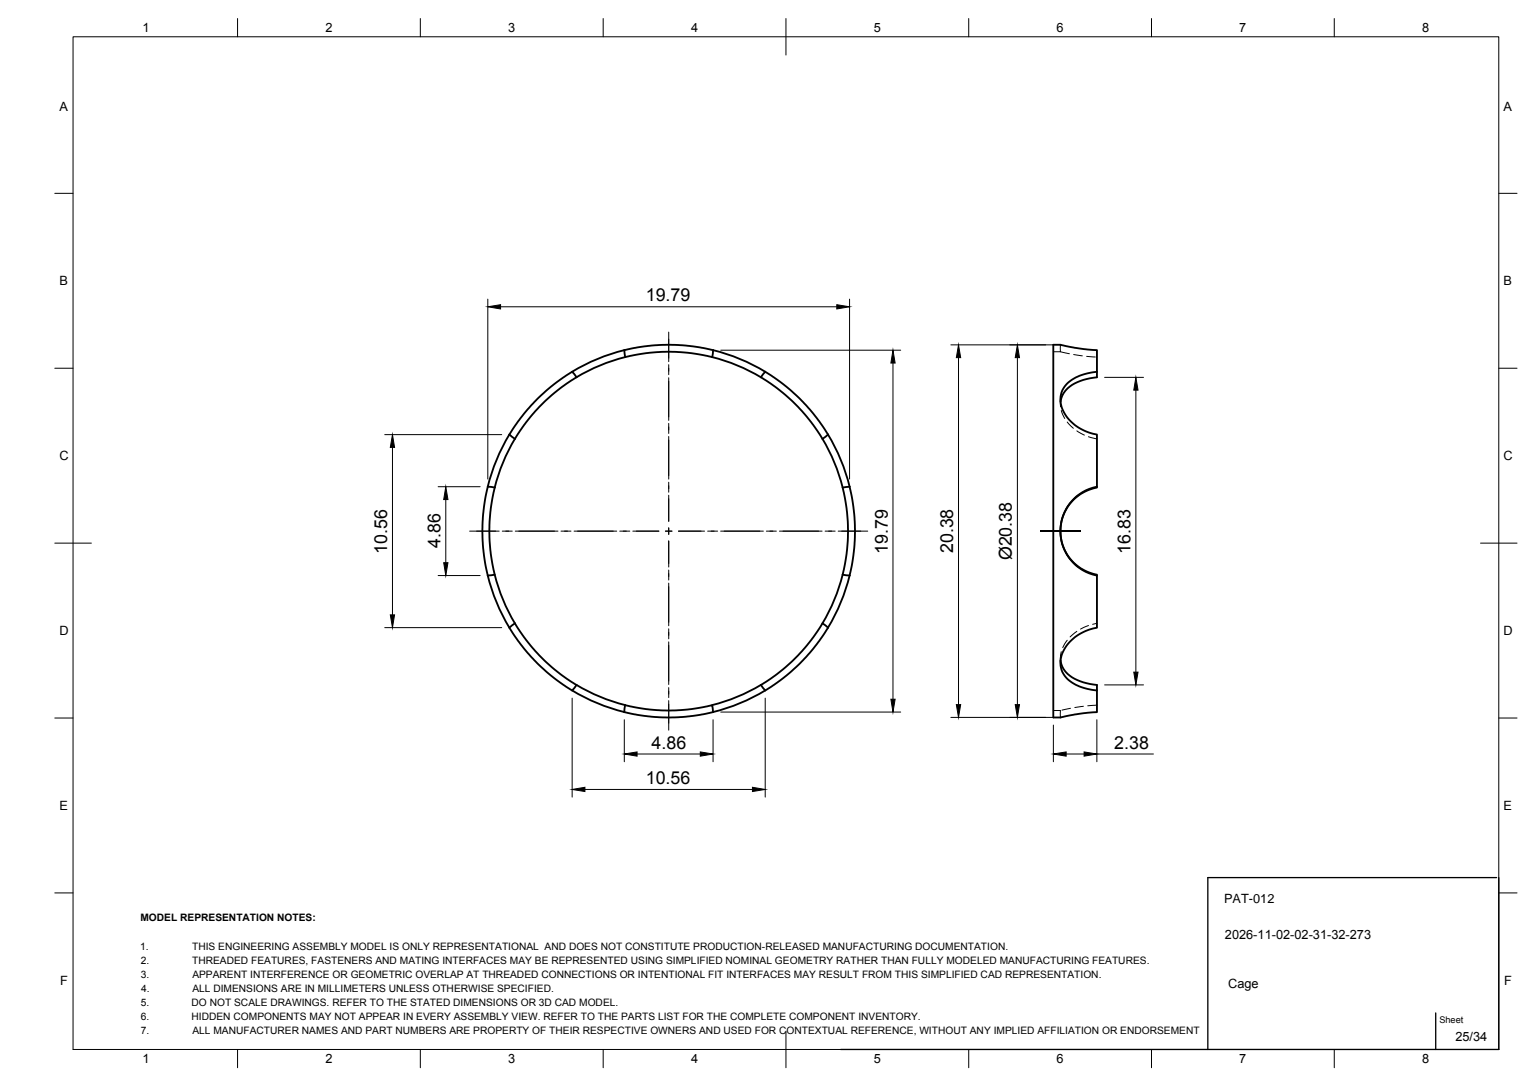
ISO-10303-21;
HEADER;
/* Generated by software containing ST-Developer
 * from STEP Tools, Inc. (www.steptools.com) 
 */

FILE_DESCRIPTION(
/* description */ ('Belt tensioner idler arm'),
/* implementation_level */ '2;1');

FILE_NAME(
/* name */ 'Cage.step',
/* time_stamp */ '2026-10-28T03:22:15-07:00',
/* author */ (''),
/* organization */ (''),
/* preprocessor_version */ 'ST-DEVELOPER v20.2',
/* originating_system */ 'Autodesk Translation Framework v15.17.0.0',
/* authorisation */ '');

FILE_SCHEMA (('AUTOMOTIVE_DESIGN { 1 0 10303 214 3 1 1 }'));
ENDSEC;

DATA;
#10=MECHANICAL_DESIGN_GEOMETRIC_PRESENTATION_REPRESENTATION('',(#475),#12779);
#263=SPHERICAL_SURFACE('',#7025,0.247676);
#264=SPHERICAL_SURFACE('',#7041,0.247676);
#265=SPHERICAL_SURFACE('',#7046,0.247676);
#266=SPHERICAL_SURFACE('',#7051,0.247676);
#267=SPHERICAL_SURFACE('',#7056,0.247676);
#268=SPHERICAL_SURFACE('',#7061,0.247676);
#269=SPHERICAL_SURFACE('',#7066,0.247676);
#270=SPHERICAL_SURFACE('',#7074,0.247676);
#334=B_SPLINE_CURVE_WITH_KNOTS('',3,(#11192,#11193,#11194,#11195,#11196,
#11197,#11198,#11199,#11200,#11201,#11202,#11203,#11204,#11205,#11206,#11207,
#11208,#11209,#11210,#11211,#11212,#11213),.UNSPECIFIED.,.F.,.F.,(4,2,2,
2,2,2,2,2,2,2,4),(0.0473477652366656,0.126350602536658,0.189525903804987,
0.252701205073317,0.313298422430275,0.373895639787233,0.434492857144191,
0.495090074501149,0.558265375769478,0.621440677037807,0.7004435143378),
 .UNSPECIFIED.);
#335=B_SPLINE_CURVE_WITH_KNOTS('',3,(#11217,#11218,#11219,#11220,#11221,
#11222,#11223,#11224,#11225,#11226,#11227,#11228,#11229,#11230,#11231,#11232,
#11233,#11234,#11235,#11236,#11237,#11238),.UNSPECIFIED.,.F.,.F.,(4,2,2,
2,2,2,2,2,2,2,4),(0.0464897534940957,0.0852567806515119,0.170513561303024,
0.246687263103517,0.308657850341199,0.370628437578881,0.432599024816563,
0.494569612054245,0.570743313854739,0.656000094506251,0.694767121663666),
 .UNSPECIFIED.);
#336=B_SPLINE_CURVE_WITH_KNOTS('',3,(#11244,#11245,#11246,#11247,#11248,
#11249,#11250,#11251,#11252,#11253,#11254,#11255,#11256,#11257,#11258,#11259,
#11260,#11261,#11262,#11263,#11264,#11265),.UNSPECIFIED.,.F.,.F.,(4,2,2,
2,2,2,2,2,2,2,4),(0.0464897534940957,0.0852567806515118,0.170513561303024,
0.246687263103517,0.308657850341199,0.370628437578881,0.432599024816563,
0.494569612054245,0.570743313854738,0.65600009450625,0.694767121663666),
 .UNSPECIFIED.);
#337=B_SPLINE_CURVE_WITH_KNOTS('',3,(#11269,#11270,#11271,#11272,#11273,
#11274,#11275,#11276,#11277,#11278,#11279,#11280,#11281,#11282,#11283,#11284,
#11285,#11286,#11287,#11288,#11289,#11290),.UNSPECIFIED.,.F.,.F.,(4,2,2,
2,2,2,2,2,2,2,4),(0.0464897534940957,0.0852567806515119,0.170513561303024,
0.246687263103517,0.308657850341199,0.370628437578881,0.432599024816563,
0.494569612054245,0.570743313854739,0.656000094506251,0.694767121663666),
 .UNSPECIFIED.);
#338=B_SPLINE_CURVE_WITH_KNOTS('',3,(#11294,#11295,#11296,#11297,#11298,
#11299,#11300,#11301,#11302,#11303,#11304,#11305),.UNSPECIFIED.,.F.,.F.,
(4,2,2,2,2,4),(0.0464897534940957,0.0852567806515119,0.170513561303024,
0.246687263103517,0.308657850341199,0.370628437578881),.UNSPECIFIED.);
#339=B_SPLINE_CURVE_WITH_KNOTS('',3,(#11310,#11311,#11312,#11313,#11314,
#11315,#11316,#11317,#11318,#11319,#11320,#11321),.UNSPECIFIED.,.F.,.F.,
(4,2,2,2,2,4),(0.370628437578881,0.432599024816563,0.494569612054245,0.570743313854738,
0.65600009450625,0.694767121663666),.UNSPECIFIED.);
#340=B_SPLINE_CURVE_WITH_KNOTS('',3,(#11325,#11326,#11327,#11328,#11329,
#11330,#11331,#11332,#11333,#11334,#11335,#11336,#11337,#11338,#11339,#11340,
#11341,#11342,#11343,#11344,#11345,#11346),.UNSPECIFIED.,.F.,.F.,(4,2,2,
2,2,2,2,2,2,2,4),(0.0464897534940957,0.0852567806515121,0.170513561303024,
0.246687263103518,0.308657850341199,0.370628437578881,0.432599024816563,
0.494569612054245,0.570743313854738,0.65600009450625,0.694767121663666),
 .UNSPECIFIED.);
#341=B_SPLINE_CURVE_WITH_KNOTS('',3,(#11350,#11351,#11352,#11353,#11354,
#11355,#11356,#11357,#11358,#11359,#11360,#11361,#11362,#11363,#11364,#11365,
#11366,#11367,#11368,#11369,#11370,#11371),.UNSPECIFIED.,.F.,.F.,(4,2,2,
2,2,2,2,2,2,2,4),(0.0464897534940957,0.0852567806515119,0.170513561303024,
0.246687263103517,0.308657850341199,0.370628437578881,0.432599024816563,
0.494569612054245,0.570743313854738,0.65600009450625,0.694767121663667),
 .UNSPECIFIED.);
#342=B_SPLINE_CURVE_WITH_KNOTS('',3,(#11375,#11376,#11377,#11378,#11379,
#11380,#11381,#11382,#11383,#11384,#11385,#11386,#11387,#11388,#11389,#11390,
#11391,#11392,#11393,#11394,#11395,#11396),.UNSPECIFIED.,.F.,.F.,(4,2,2,
2,2,2,2,2,2,2,4),(0.0464897534940957,0.0852567806515119,0.170513561303024,
0.246687263103517,0.308657850341199,0.370628437578881,0.432599024816563,
0.494569612054245,0.570743313854738,0.65600009450625,0.694767121663666),
 .UNSPECIFIED.);
#343=B_SPLINE_CURVE_WITH_KNOTS('',3,(#11400,#11401,#11402,#11403,#11404,
#11405,#11406,#11407,#11408,#11409,#11410,#11411,#11412,#11413,#11414,#11415,
#11416,#11417,#11418,#11419,#11420,#11421),.UNSPECIFIED.,.F.,.F.,(4,2,2,
2,2,2,2,2,2,2,4),(0.0464897534940957,0.0852567806515119,0.170513561303024,
0.246687263103517,0.308657850341199,0.370628437578881,0.432599024816563,
0.494569612054245,0.570743313854739,0.656000094506251,0.694767121663667),
 .UNSPECIFIED.);
#344=B_SPLINE_CURVE_WITH_KNOTS('',3,(#11429,#11430,#11431,#11432,#11433,
#11434,#11435,#11436,#11437,#11438,#11439,#11440,#11441,#11442,#11443,#11444,
#11445,#11446,#11447,#11448,#11449,#11450),.UNSPECIFIED.,.F.,.F.,(4,2,2,
2,2,2,2,2,2,2,4),(0.0473477652366656,0.126350602536658,0.189525903804987,
0.252701205073316,0.313298422430274,0.373895639787232,0.434492857144191,
0.495090074501149,0.558265375769478,0.621440677037807,0.7004435143378),
 .UNSPECIFIED.);
#345=B_SPLINE_CURVE_WITH_KNOTS('',3,(#11458,#11459,#11460,#11461,#11462,
#11463,#11464,#11465,#11466,#11467,#11468,#11469,#11470,#11471,#11472,#11473,
#11474,#11475,#11476,#11477,#11478,#11479),.UNSPECIFIED.,.F.,.F.,(4,2,2,
2,2,2,2,2,2,2,4),(0.0473477652366656,0.126350602536658,0.189525903804987,
0.252701205073317,0.313298422430275,0.373895639787233,0.434492857144191,
0.495090074501149,0.558265375769478,0.621440677037807,0.7004435143378),
 .UNSPECIFIED.);
#346=B_SPLINE_CURVE_WITH_KNOTS('',3,(#11488,#11489,#11490,#11491,#11492,
#11493,#11494,#11495,#11496,#11497,#11498,#11499),.UNSPECIFIED.,.F.,.F.,
(4,2,2,2,2,4),(0.0473477652366656,0.126350602536658,0.189525903804987,0.252701205073316,
0.313298422430275,0.373895639787233),.UNSPECIFIED.);
#347=B_SPLINE_CURVE_WITH_KNOTS('',3,(#11501,#11502,#11503,#11504,#11505,
#11506,#11507,#11508,#11509,#11510,#11511,#11512),.UNSPECIFIED.,.F.,.F.,
(4,2,2,2,2,4),(0.373895639787233,0.434492857144191,0.495090074501149,0.558265375769478,
0.621440677037807,0.7004435143378),.UNSPECIFIED.);
#348=B_SPLINE_CURVE_WITH_KNOTS('',3,(#11519,#11520,#11521,#11522,#11523,
#11524,#11525,#11526,#11527,#11528,#11529,#11530,#11531,#11532,#11533,#11534,
#11535,#11536,#11537,#11538,#11539,#11540),.UNSPECIFIED.,.F.,.F.,(4,2,2,
2,2,2,2,2,2,2,4),(0.0473477652366656,0.126350602536658,0.189525903804987,
0.252701205073316,0.313298422430275,0.373895639787233,0.434492857144191,
0.495090074501149,0.558265375769478,0.621440677037807,0.7004435143378),
 .UNSPECIFIED.);
#349=B_SPLINE_CURVE_WITH_KNOTS('',3,(#11548,#11549,#11550,#11551,#11552,
#11553,#11554,#11555,#11556,#11557,#11558,#11559,#11560,#11561,#11562,#11563,
#11564,#11565,#11566,#11567,#11568,#11569),.UNSPECIFIED.,.F.,.F.,(4,2,2,
2,2,2,2,2,2,2,4),(0.0473477652366656,0.126350602536658,0.189525903804987,
0.252701205073317,0.313298422430275,0.373895639787233,0.434492857144191,
0.495090074501149,0.558265375769478,0.621440677037807,0.7004435143378),
 .UNSPECIFIED.);
#350=B_SPLINE_CURVE_WITH_KNOTS('',3,(#11577,#11578,#11579,#11580,#11581,
#11582,#11583,#11584,#11585,#11586,#11587,#11588,#11589,#11590,#11591,#11592,
#11593,#11594,#11595,#11596,#11597,#11598),.UNSPECIFIED.,.F.,.F.,(4,2,2,
2,2,2,2,2,2,2,4),(0.0473477652366656,0.126350602536658,0.189525903804987,
0.252701205073316,0.313298422430275,0.373895639787233,0.434492857144191,
0.495090074501149,0.558265375769478,0.621440677037807,0.7004435143378),
 .UNSPECIFIED.);
#351=B_SPLINE_CURVE_WITH_KNOTS('',3,(#11607,#11608,#11609,#11610,#11611,
#11612,#11613,#11614,#11615,#11616,#11617,#11618,#11619,#11620,#11621,#11622,
#11623,#11624,#11625,#11626,#11627,#11628),.UNSPECIFIED.,.F.,.F.,(4,2,2,
2,2,2,2,2,2,2,4),(0.0473477652366656,0.126350602536658,0.189525903804987,
0.252701205073317,0.313298422430275,0.373895639787233,0.434492857144191,
0.495090074501149,0.558265375769478,0.621440677037807,0.7004435143378),
 .UNSPECIFIED.);
#400=SHAPE_REPRESENTATION_RELATIONSHIP('SRR','None',#12948,#434);
#434=ADVANCED_BREP_SHAPE_REPRESENTATION('',(#515),#12765);
#475=STYLED_ITEM('',(#13184),#515);
#515=MANIFOLD_SOLID_BREP('Continuous crown cage',#6211);
#631=FACE_BOUND('',#1536,.T.);
#769=PLANE('',#7038);
#770=PLANE('',#7043);
#771=PLANE('',#7048);
#772=PLANE('',#7053);
#773=PLANE('',#7058);
#774=PLANE('',#7063);
#775=PLANE('',#7072);
#776=PLANE('',#7076);
#777=PLANE('',#7077);
#1047=FACE_OUTER_BOUND('',#1518,.T.);
#1048=FACE_OUTER_BOUND('',#1519,.T.);
#1049=FACE_OUTER_BOUND('',#1520,.T.);
#1050=FACE_OUTER_BOUND('',#1521,.T.);
#1051=FACE_OUTER_BOUND('',#1522,.T.);
#1052=FACE_OUTER_BOUND('',#1523,.T.);
#1053=FACE_OUTER_BOUND('',#1524,.T.);
#1054=FACE_OUTER_BOUND('',#1525,.T.);
#1055=FACE_OUTER_BOUND('',#1526,.T.);
#1056=FACE_OUTER_BOUND('',#1527,.T.);
#1057=FACE_OUTER_BOUND('',#1528,.T.);
#1058=FACE_OUTER_BOUND('',#1529,.T.);
#1059=FACE_OUTER_BOUND('',#1530,.T.);
#1060=FACE_OUTER_BOUND('',#1531,.T.);
#1061=FACE_OUTER_BOUND('',#1532,.T.);
#1062=FACE_OUTER_BOUND('',#1533,.T.);
#1063=FACE_OUTER_BOUND('',#1534,.T.);
#1064=FACE_OUTER_BOUND('',#1535,.T.);
#1065=FACE_OUTER_BOUND('',#1537,.T.);
#1518=EDGE_LOOP('',(#4940,#4941,#4942,#4943));
#1519=EDGE_LOOP('',(#4944,#4945,#4946,#4947,#4948,#4949,#4950,#4951,#4952,
#4953,#4954,#4955,#4956,#4957,#4958,#4959,#4960,#4961,#4962,#4963));
#1520=EDGE_LOOP('',(#4964,#4965,#4966,#4967));
#1521=EDGE_LOOP('',(#4968,#4969,#4970,#4971));
#1522=EDGE_LOOP('',(#4972,#4973,#4974,#4975));
#1523=EDGE_LOOP('',(#4976,#4977,#4978,#4979));
#1524=EDGE_LOOP('',(#4980,#4981,#4982,#4983));
#1525=EDGE_LOOP('',(#4984,#4985,#4986,#4987,#4988,#4989));
#1526=EDGE_LOOP('',(#4990,#4991,#4992,#4993));
#1527=EDGE_LOOP('',(#4994,#4995,#4996,#4997));
#1528=EDGE_LOOP('',(#4998,#4999,#5000,#5001));
#1529=EDGE_LOOP('',(#5002,#5003,#5004,#5005));
#1530=EDGE_LOOP('',(#5006,#5007,#5008,#5009));
#1531=EDGE_LOOP('',(#5010,#5011,#5012,#5013));
#1532=EDGE_LOOP('',(#5014,#5015,#5016,#5017,#5018,#5019,#5020,#5021,#5022,
#5023,#5024,#5025,#5026,#5027,#5028,#5029,#5030,#5031,#5032,#5033));
#1533=EDGE_LOOP('',(#5034,#5035,#5036,#5037));
#1534=EDGE_LOOP('',(#5038,#5039,#5040,#5041));
#1535=EDGE_LOOP('',(#5042));
#1536=EDGE_LOOP('',(#5043));
#1537=EDGE_LOOP('',(#5044,#5045,#5046,#5047));
#1917=LINE('',#11307,#2266);
#1918=LINE('',#11603,#2267);
#2266=VECTOR('',#8503,1.019052);
#2267=VECTOR('',#8580,0.980948);
#2592=CIRCLE('',#7026,0.243053047864041);
#2593=CIRCLE('',#7027,0.243053047864041);
#2594=CIRCLE('',#7029,1.019052);
#2595=CIRCLE('',#7030,1.019052);
#2596=CIRCLE('',#7031,1.019052);
#2597=CIRCLE('',#7032,1.019052);
#2598=CIRCLE('',#7033,1.019052);
#2599=CIRCLE('',#7034,1.019052);
#2600=CIRCLE('',#7035,1.019052);
#2601=CIRCLE('',#7036,1.019052);
#2602=CIRCLE('',#7037,1.019052);
#2603=CIRCLE('',#7039,0.980948);
#2604=CIRCLE('',#7040,0.243053047864041);
#2605=CIRCLE('',#7042,0.243053047864041);
#2606=CIRCLE('',#7044,0.980948);
#2607=CIRCLE('',#7045,0.243053047864041);
#2608=CIRCLE('',#7047,0.243053047864041);
#2609=CIRCLE('',#7049,0.980948);
#2610=CIRCLE('',#7050,0.243053047864041);
#2611=CIRCLE('',#7052,0.243053047864041);
#2612=CIRCLE('',#7054,0.980948);
#2613=CIRCLE('',#7055,0.243053047864041);
#2614=CIRCLE('',#7057,0.243053047864041);
#2615=CIRCLE('',#7059,0.980948);
#2616=CIRCLE('',#7060,0.243053047864041);
#2617=CIRCLE('',#7062,0.243053047864041);
#2618=CIRCLE('',#7064,0.980948);
#2619=CIRCLE('',#7065,0.243053047864041);
#2620=CIRCLE('',#7067,0.243053047864041);
#2621=CIRCLE('',#7069,0.980948);
#2622=CIRCLE('',#7070,0.980948);
#2623=CIRCLE('',#7071,0.980948);
#2624=CIRCLE('',#7073,0.243053047864041);
#2625=CIRCLE('',#7075,0.243053047864041);
#3056=VERTEX_POINT('',#11190);
#3057=VERTEX_POINT('',#11191);
#3058=VERTEX_POINT('',#11214);
#3059=VERTEX_POINT('',#11216);
#3060=VERTEX_POINT('',#11241);
#3061=VERTEX_POINT('',#11243);
#3062=VERTEX_POINT('',#11266);
#3063=VERTEX_POINT('',#11268);
#3064=VERTEX_POINT('',#11291);
#3065=VERTEX_POINT('',#11293);
#3066=VERTEX_POINT('',#11306);
#3067=VERTEX_POINT('',#11309);
#3068=VERTEX_POINT('',#11322);
#3069=VERTEX_POINT('',#11324);
#3070=VERTEX_POINT('',#11347);
#3071=VERTEX_POINT('',#11349);
#3072=VERTEX_POINT('',#11372);
#3073=VERTEX_POINT('',#11374);
#3074=VERTEX_POINT('',#11397);
#3075=VERTEX_POINT('',#11399);
#3076=VERTEX_POINT('',#11424);
#3077=VERTEX_POINT('',#11428);
#3078=VERTEX_POINT('',#11453);
#3079=VERTEX_POINT('',#11457);
#3080=VERTEX_POINT('',#11482);
#3081=VERTEX_POINT('',#11486);
#3082=VERTEX_POINT('',#11487);
#3083=VERTEX_POINT('',#11514);
#3084=VERTEX_POINT('',#11518);
#3085=VERTEX_POINT('',#11543);
#3086=VERTEX_POINT('',#11547);
#3087=VERTEX_POINT('',#11572);
#3088=VERTEX_POINT('',#11576);
#3089=VERTEX_POINT('',#11601);
#3090=VERTEX_POINT('',#11604);
#3091=VERTEX_POINT('',#11606);
#3725=EDGE_CURVE('',#3056,#3057,#334,.T.);
#3726=EDGE_CURVE('',#3058,#3056,#2592,.T.);
#3727=EDGE_CURVE('',#3059,#3058,#335,.T.);
#3728=EDGE_CURVE('',#3057,#3059,#2593,.T.);
#3729=EDGE_CURVE('',#3060,#3058,#2594,.T.);
#3730=EDGE_CURVE('',#3060,#3061,#336,.T.);
#3731=EDGE_CURVE('',#3062,#3061,#2595,.T.);
#3732=EDGE_CURVE('',#3062,#3063,#337,.T.);
#3733=EDGE_CURVE('',#3064,#3063,#2596,.T.);
#3734=EDGE_CURVE('',#3064,#3065,#338,.T.);
#3735=EDGE_CURVE('',#3065,#3066,#1917,.T.);
#3736=EDGE_CURVE('',#3066,#3066,#2597,.T.);
#3737=EDGE_CURVE('',#3065,#3067,#339,.T.);
#3738=EDGE_CURVE('',#3068,#3067,#2598,.T.);
#3739=EDGE_CURVE('',#3068,#3069,#340,.T.);
#3740=EDGE_CURVE('',#3070,#3069,#2599,.T.);
#3741=EDGE_CURVE('',#3070,#3071,#341,.T.);
#3742=EDGE_CURVE('',#3072,#3071,#2600,.T.);
#3743=EDGE_CURVE('',#3072,#3073,#342,.T.);
#3744=EDGE_CURVE('',#3074,#3073,#2601,.T.);
#3745=EDGE_CURVE('',#3074,#3075,#343,.T.);
#3746=EDGE_CURVE('',#3059,#3075,#2602,.T.);
#3747=EDGE_CURVE('',#3056,#3076,#2603,.T.);
#3748=EDGE_CURVE('',#3076,#3060,#2604,.T.);
#3749=EDGE_CURVE('',#3077,#3076,#344,.T.);
#3750=EDGE_CURVE('',#3061,#3077,#2605,.T.);
#3751=EDGE_CURVE('',#3077,#3078,#2606,.T.);
#3752=EDGE_CURVE('',#3078,#3062,#2607,.T.);
#3753=EDGE_CURVE('',#3079,#3078,#345,.T.);
#3754=EDGE_CURVE('',#3063,#3079,#2608,.T.);
#3755=EDGE_CURVE('',#3079,#3080,#2609,.T.);
#3756=EDGE_CURVE('',#3080,#3064,#2610,.T.);
#3757=EDGE_CURVE('',#3081,#3082,#346,.T.);
#3758=EDGE_CURVE('',#3067,#3081,#2611,.T.);
#3759=EDGE_CURVE('',#3082,#3080,#347,.T.);
#3760=EDGE_CURVE('',#3081,#3083,#2612,.T.);
#3761=EDGE_CURVE('',#3083,#3068,#2613,.T.);
#3762=EDGE_CURVE('',#3084,#3083,#348,.T.);
#3763=EDGE_CURVE('',#3069,#3084,#2614,.T.);
#3764=EDGE_CURVE('',#3084,#3085,#2615,.T.);
#3765=EDGE_CURVE('',#3085,#3070,#2616,.T.);
#3766=EDGE_CURVE('',#3086,#3085,#349,.T.);
#3767=EDGE_CURVE('',#3071,#3086,#2617,.T.);
#3768=EDGE_CURVE('',#3086,#3087,#2618,.T.);
#3769=EDGE_CURVE('',#3087,#3072,#2619,.T.);
#3770=EDGE_CURVE('',#3088,#3087,#350,.T.);
#3771=EDGE_CURVE('',#3073,#3088,#2620,.T.);
#3772=EDGE_CURVE('',#3089,#3089,#2621,.T.);
#3773=EDGE_CURVE('',#3089,#3082,#1918,.T.);
#3774=EDGE_CURVE('',#3090,#3057,#2622,.T.);
#3775=EDGE_CURVE('',#3090,#3091,#351,.T.);
#3776=EDGE_CURVE('',#3088,#3091,#2623,.T.);
#3777=EDGE_CURVE('',#3075,#3090,#2624,.T.);
#3778=EDGE_CURVE('',#3091,#3074,#2625,.T.);
#4940=ORIENTED_EDGE('',*,*,#3725,.F.);
#4941=ORIENTED_EDGE('',*,*,#3726,.F.);
#4942=ORIENTED_EDGE('',*,*,#3727,.F.);
#4943=ORIENTED_EDGE('',*,*,#3728,.F.);
#4944=ORIENTED_EDGE('',*,*,#3727,.T.);
#4945=ORIENTED_EDGE('',*,*,#3729,.F.);
#4946=ORIENTED_EDGE('',*,*,#3730,.T.);
#4947=ORIENTED_EDGE('',*,*,#3731,.F.);
#4948=ORIENTED_EDGE('',*,*,#3732,.T.);
#4949=ORIENTED_EDGE('',*,*,#3733,.F.);
#4950=ORIENTED_EDGE('',*,*,#3734,.T.);
#4951=ORIENTED_EDGE('',*,*,#3735,.T.);
#4952=ORIENTED_EDGE('',*,*,#3736,.F.);
#4953=ORIENTED_EDGE('',*,*,#3735,.F.);
#4954=ORIENTED_EDGE('',*,*,#3737,.T.);
#4955=ORIENTED_EDGE('',*,*,#3738,.F.);
#4956=ORIENTED_EDGE('',*,*,#3739,.T.);
#4957=ORIENTED_EDGE('',*,*,#3740,.F.);
#4958=ORIENTED_EDGE('',*,*,#3741,.T.);
#4959=ORIENTED_EDGE('',*,*,#3742,.F.);
#4960=ORIENTED_EDGE('',*,*,#3743,.T.);
#4961=ORIENTED_EDGE('',*,*,#3744,.F.);
#4962=ORIENTED_EDGE('',*,*,#3745,.T.);
#4963=ORIENTED_EDGE('',*,*,#3746,.F.);
#4964=ORIENTED_EDGE('',*,*,#3726,.T.);
#4965=ORIENTED_EDGE('',*,*,#3747,.T.);
#4966=ORIENTED_EDGE('',*,*,#3748,.T.);
#4967=ORIENTED_EDGE('',*,*,#3729,.T.);
#4968=ORIENTED_EDGE('',*,*,#3749,.F.);
#4969=ORIENTED_EDGE('',*,*,#3750,.F.);
#4970=ORIENTED_EDGE('',*,*,#3730,.F.);
#4971=ORIENTED_EDGE('',*,*,#3748,.F.);
#4972=ORIENTED_EDGE('',*,*,#3750,.T.);
#4973=ORIENTED_EDGE('',*,*,#3751,.T.);
#4974=ORIENTED_EDGE('',*,*,#3752,.T.);
#4975=ORIENTED_EDGE('',*,*,#3731,.T.);
#4976=ORIENTED_EDGE('',*,*,#3753,.F.);
#4977=ORIENTED_EDGE('',*,*,#3754,.F.);
#4978=ORIENTED_EDGE('',*,*,#3732,.F.);
#4979=ORIENTED_EDGE('',*,*,#3752,.F.);
#4980=ORIENTED_EDGE('',*,*,#3754,.T.);
#4981=ORIENTED_EDGE('',*,*,#3755,.T.);
#4982=ORIENTED_EDGE('',*,*,#3756,.T.);
#4983=ORIENTED_EDGE('',*,*,#3733,.T.);
#4984=ORIENTED_EDGE('',*,*,#3757,.F.);
#4985=ORIENTED_EDGE('',*,*,#3758,.F.);
#4986=ORIENTED_EDGE('',*,*,#3737,.F.);
#4987=ORIENTED_EDGE('',*,*,#3734,.F.);
#4988=ORIENTED_EDGE('',*,*,#3756,.F.);
#4989=ORIENTED_EDGE('',*,*,#3759,.F.);
#4990=ORIENTED_EDGE('',*,*,#3758,.T.);
#4991=ORIENTED_EDGE('',*,*,#3760,.T.);
#4992=ORIENTED_EDGE('',*,*,#3761,.T.);
#4993=ORIENTED_EDGE('',*,*,#3738,.T.);
#4994=ORIENTED_EDGE('',*,*,#3762,.F.);
#4995=ORIENTED_EDGE('',*,*,#3763,.F.);
#4996=ORIENTED_EDGE('',*,*,#3739,.F.);
#4997=ORIENTED_EDGE('',*,*,#3761,.F.);
#4998=ORIENTED_EDGE('',*,*,#3763,.T.);
#4999=ORIENTED_EDGE('',*,*,#3764,.T.);
#5000=ORIENTED_EDGE('',*,*,#3765,.T.);
#5001=ORIENTED_EDGE('',*,*,#3740,.T.);
#5002=ORIENTED_EDGE('',*,*,#3766,.F.);
#5003=ORIENTED_EDGE('',*,*,#3767,.F.);
#5004=ORIENTED_EDGE('',*,*,#3741,.F.);
#5005=ORIENTED_EDGE('',*,*,#3765,.F.);
#5006=ORIENTED_EDGE('',*,*,#3767,.T.);
#5007=ORIENTED_EDGE('',*,*,#3768,.T.);
#5008=ORIENTED_EDGE('',*,*,#3769,.T.);
#5009=ORIENTED_EDGE('',*,*,#3742,.T.);
#5010=ORIENTED_EDGE('',*,*,#3743,.F.);
#5011=ORIENTED_EDGE('',*,*,#3769,.F.);
#5012=ORIENTED_EDGE('',*,*,#3770,.F.);
#5013=ORIENTED_EDGE('',*,*,#3771,.F.);
#5014=ORIENTED_EDGE('',*,*,#3772,.F.);
#5015=ORIENTED_EDGE('',*,*,#3773,.T.);
#5016=ORIENTED_EDGE('',*,*,#3759,.T.);
#5017=ORIENTED_EDGE('',*,*,#3755,.F.);
#5018=ORIENTED_EDGE('',*,*,#3753,.T.);
#5019=ORIENTED_EDGE('',*,*,#3751,.F.);
#5020=ORIENTED_EDGE('',*,*,#3749,.T.);
#5021=ORIENTED_EDGE('',*,*,#3747,.F.);
#5022=ORIENTED_EDGE('',*,*,#3725,.T.);
#5023=ORIENTED_EDGE('',*,*,#3774,.F.);
#5024=ORIENTED_EDGE('',*,*,#3775,.T.);
#5025=ORIENTED_EDGE('',*,*,#3776,.F.);
#5026=ORIENTED_EDGE('',*,*,#3770,.T.);
#5027=ORIENTED_EDGE('',*,*,#3768,.F.);
#5028=ORIENTED_EDGE('',*,*,#3766,.T.);
#5029=ORIENTED_EDGE('',*,*,#3764,.F.);
#5030=ORIENTED_EDGE('',*,*,#3762,.T.);
#5031=ORIENTED_EDGE('',*,*,#3760,.F.);
#5032=ORIENTED_EDGE('',*,*,#3757,.T.);
#5033=ORIENTED_EDGE('',*,*,#3773,.F.);
#5034=ORIENTED_EDGE('',*,*,#3728,.T.);
#5035=ORIENTED_EDGE('',*,*,#3746,.T.);
#5036=ORIENTED_EDGE('',*,*,#3777,.T.);
#5037=ORIENTED_EDGE('',*,*,#3774,.T.);
#5038=ORIENTED_EDGE('',*,*,#3745,.F.);
#5039=ORIENTED_EDGE('',*,*,#3778,.F.);
#5040=ORIENTED_EDGE('',*,*,#3775,.F.);
#5041=ORIENTED_EDGE('',*,*,#3777,.F.);
#5042=ORIENTED_EDGE('',*,*,#3736,.T.);
#5043=ORIENTED_EDGE('',*,*,#3772,.T.);
#5044=ORIENTED_EDGE('',*,*,#3771,.T.);
#5045=ORIENTED_EDGE('',*,*,#3776,.T.);
#5046=ORIENTED_EDGE('',*,*,#3778,.T.);
#5047=ORIENTED_EDGE('',*,*,#3744,.T.);
#5740=CYLINDRICAL_SURFACE('',#7028,1.019052);
#5741=CYLINDRICAL_SURFACE('',#7068,0.980948);
#6024=ADVANCED_FACE('',(#1047),#263,.F.);
#6025=ADVANCED_FACE('',(#1048),#5740,.T.);
#6026=ADVANCED_FACE('',(#1049),#769,.T.);
#6027=ADVANCED_FACE('',(#1050),#264,.F.);
#6028=ADVANCED_FACE('',(#1051),#770,.T.);
#6029=ADVANCED_FACE('',(#1052),#265,.F.);
#6030=ADVANCED_FACE('',(#1053),#771,.T.);
#6031=ADVANCED_FACE('',(#1054),#266,.F.);
#6032=ADVANCED_FACE('',(#1055),#772,.T.);
#6033=ADVANCED_FACE('',(#1056),#267,.F.);
#6034=ADVANCED_FACE('',(#1057),#773,.T.);
#6035=ADVANCED_FACE('',(#1058),#268,.F.);
#6036=ADVANCED_FACE('',(#1059),#774,.T.);
#6037=ADVANCED_FACE('',(#1060),#269,.F.);
#6038=ADVANCED_FACE('',(#1061),#5741,.F.);
#6039=ADVANCED_FACE('',(#1062),#775,.T.);
#6040=ADVANCED_FACE('',(#1063),#270,.F.);
#6041=ADVANCED_FACE('',(#1064,#631),#776,.T.);
#6042=ADVANCED_FACE('',(#1065),#777,.T.);
#6211=CLOSED_SHELL('',(#6024,#6025,#6026,#6027,#6028,#6029,#6030,#6031,
#6032,#6033,#6034,#6035,#6036,#6037,#6038,#6039,#6040,#6041,#6042));
#7024=AXIS2_PLACEMENT_3D('',#11188,#8487,#8488);
#7025=AXIS2_PLACEMENT_3D('',#11189,#8489,#8490);
#7026=AXIS2_PLACEMENT_3D('',#11215,#8491,#8492);
#7027=AXIS2_PLACEMENT_3D('',#11239,#8493,#8494);
#7028=AXIS2_PLACEMENT_3D('',#11240,#8495,#8496);
#7029=AXIS2_PLACEMENT_3D('',#11242,#8497,#8498);
#7030=AXIS2_PLACEMENT_3D('',#11267,#8499,#8500);
#7031=AXIS2_PLACEMENT_3D('',#11292,#8501,#8502);
#7032=AXIS2_PLACEMENT_3D('',#11308,#8504,#8505);
#7033=AXIS2_PLACEMENT_3D('',#11323,#8506,#8507);
#7034=AXIS2_PLACEMENT_3D('',#11348,#8508,#8509);
#7035=AXIS2_PLACEMENT_3D('',#11373,#8510,#8511);
#7036=AXIS2_PLACEMENT_3D('',#11398,#8512,#8513);
#7037=AXIS2_PLACEMENT_3D('',#11422,#8514,#8515);
#7038=AXIS2_PLACEMENT_3D('',#11423,#8516,#8517);
#7039=AXIS2_PLACEMENT_3D('',#11425,#8518,#8519);
#7040=AXIS2_PLACEMENT_3D('',#11426,#8520,#8521);
#7041=AXIS2_PLACEMENT_3D('',#11427,#8522,#8523);
#7042=AXIS2_PLACEMENT_3D('',#11451,#8524,#8525);
#7043=AXIS2_PLACEMENT_3D('',#11452,#8526,#8527);
#7044=AXIS2_PLACEMENT_3D('',#11454,#8528,#8529);
#7045=AXIS2_PLACEMENT_3D('',#11455,#8530,#8531);
#7046=AXIS2_PLACEMENT_3D('',#11456,#8532,#8533);
#7047=AXIS2_PLACEMENT_3D('',#11480,#8534,#8535);
#7048=AXIS2_PLACEMENT_3D('',#11481,#8536,#8537);
#7049=AXIS2_PLACEMENT_3D('',#11483,#8538,#8539);
#7050=AXIS2_PLACEMENT_3D('',#11484,#8540,#8541);
#7051=AXIS2_PLACEMENT_3D('',#11485,#8542,#8543);
#7052=AXIS2_PLACEMENT_3D('',#11500,#8544,#8545);
#7053=AXIS2_PLACEMENT_3D('',#11513,#8546,#8547);
#7054=AXIS2_PLACEMENT_3D('',#11515,#8548,#8549);
#7055=AXIS2_PLACEMENT_3D('',#11516,#8550,#8551);
#7056=AXIS2_PLACEMENT_3D('',#11517,#8552,#8553);
#7057=AXIS2_PLACEMENT_3D('',#11541,#8554,#8555);
#7058=AXIS2_PLACEMENT_3D('',#11542,#8556,#8557);
#7059=AXIS2_PLACEMENT_3D('',#11544,#8558,#8559);
#7060=AXIS2_PLACEMENT_3D('',#11545,#8560,#8561);
#7061=AXIS2_PLACEMENT_3D('',#11546,#8562,#8563);
#7062=AXIS2_PLACEMENT_3D('',#11570,#8564,#8565);
#7063=AXIS2_PLACEMENT_3D('',#11571,#8566,#8567);
#7064=AXIS2_PLACEMENT_3D('',#11573,#8568,#8569);
#7065=AXIS2_PLACEMENT_3D('',#11574,#8570,#8571);
#7066=AXIS2_PLACEMENT_3D('',#11575,#8572,#8573);
#7067=AXIS2_PLACEMENT_3D('',#11599,#8574,#8575);
#7068=AXIS2_PLACEMENT_3D('',#11600,#8576,#8577);
#7069=AXIS2_PLACEMENT_3D('',#11602,#8578,#8579);
#7070=AXIS2_PLACEMENT_3D('',#11605,#8581,#8582);
#7071=AXIS2_PLACEMENT_3D('',#11629,#8583,#8584);
#7072=AXIS2_PLACEMENT_3D('',#11630,#8585,#8586);
#7073=AXIS2_PLACEMENT_3D('',#11631,#8587,#8588);
#7074=AXIS2_PLACEMENT_3D('',#11632,#8589,#8590);
#7075=AXIS2_PLACEMENT_3D('',#11633,#8591,#8592);
#7076=AXIS2_PLACEMENT_3D('',#11634,#8593,#8594);
#7077=AXIS2_PLACEMENT_3D('',#11635,#8595,#8596);
#8487=DIRECTION('axis',(0.,0.,1.));
#8488=DIRECTION('refdir',(1.,0.,0.));
#8489=DIRECTION('center_axis',(0.,0.,1.));
#8490=DIRECTION('ref_axis',(1.,0.,0.));
#8491=DIRECTION('center_axis',(0.,-1.,0.));
#8492=DIRECTION('ref_axis',(0.,0.,-1.));
#8493=DIRECTION('center_axis',(0.,-1.,0.));
#8494=DIRECTION('ref_axis',(0.,0.,-1.));
#8495=DIRECTION('center_axis',(0.,1.,0.));
#8496=DIRECTION('ref_axis',(1.,0.,0.));
#8497=DIRECTION('center_axis',(0.,1.,0.));
#8498=DIRECTION('ref_axis',(1.,0.,0.));
#8499=DIRECTION('center_axis',(0.,1.,0.));
#8500=DIRECTION('ref_axis',(1.,0.,0.));
#8501=DIRECTION('center_axis',(0.,1.,0.));
#8502=DIRECTION('ref_axis',(1.,0.,0.));
#8503=DIRECTION('',(0.,-1.,0.));
#8504=DIRECTION('center_axis',(0.,-1.,0.));
#8505=DIRECTION('ref_axis',(1.,0.,0.));
#8506=DIRECTION('center_axis',(0.,1.,0.));
#8507=DIRECTION('ref_axis',(1.,0.,0.));
#8508=DIRECTION('center_axis',(0.,1.,0.));
#8509=DIRECTION('ref_axis',(1.,0.,0.));
#8510=DIRECTION('center_axis',(0.,1.,0.));
#8511=DIRECTION('ref_axis',(1.,0.,0.));
#8512=DIRECTION('center_axis',(0.,1.,0.));
#8513=DIRECTION('ref_axis',(1.,0.,0.));
#8514=DIRECTION('center_axis',(0.,1.,0.));
#8515=DIRECTION('ref_axis',(1.,0.,0.));
#8516=DIRECTION('center_axis',(0.,1.,0.));
#8517=DIRECTION('ref_axis',(1.,0.,0.));
#8518=DIRECTION('center_axis',(0.,-1.,0.));
#8519=DIRECTION('ref_axis',(1.,0.,0.));
#8520=DIRECTION('center_axis',(0.,-1.,0.));
#8521=DIRECTION('ref_axis',(0.,0.,-1.));
#8522=DIRECTION('center_axis',(6.12323399573677E-17,0.,1.));
#8523=DIRECTION('ref_axis',(1.,0.,0.));
#8524=DIRECTION('center_axis',(0.,-1.,0.));
#8525=DIRECTION('ref_axis',(0.,0.,-1.));
#8526=DIRECTION('center_axis',(0.,1.,0.));
#8527=DIRECTION('ref_axis',(1.,0.,0.));
#8528=DIRECTION('center_axis',(0.,-1.,0.));
#8529=DIRECTION('ref_axis',(1.,0.,0.));
#8530=DIRECTION('center_axis',(0.,-1.,0.));
#8531=DIRECTION('ref_axis',(0.,0.,-1.));
#8532=DIRECTION('center_axis',(0.,0.,1.));
#8533=DIRECTION('ref_axis',(1.,0.,0.));
#8534=DIRECTION('center_axis',(0.,-1.,0.));
#8535=DIRECTION('ref_axis',(0.,0.,-1.));
#8536=DIRECTION('center_axis',(0.,1.,0.));
#8537=DIRECTION('ref_axis',(1.,0.,0.));
#8538=DIRECTION('center_axis',(0.,-1.,0.));
#8539=DIRECTION('ref_axis',(1.,0.,0.));
#8540=DIRECTION('center_axis',(0.,-1.,0.));
#8541=DIRECTION('ref_axis',(0.,0.,-1.));
#8542=DIRECTION('center_axis',(0.,0.,1.));
#8543=DIRECTION('ref_axis',(1.,0.,0.));
#8544=DIRECTION('center_axis',(0.,-1.,0.));
#8545=DIRECTION('ref_axis',(0.,0.,-1.));
#8546=DIRECTION('center_axis',(0.,1.,0.));
#8547=DIRECTION('ref_axis',(1.,0.,0.));
#8548=DIRECTION('center_axis',(0.,-1.,0.));
#8549=DIRECTION('ref_axis',(1.,0.,0.));
#8550=DIRECTION('center_axis',(0.,-1.,0.));
#8551=DIRECTION('ref_axis',(0.,0.,-1.));
#8552=DIRECTION('center_axis',(0.,0.,1.));
#8553=DIRECTION('ref_axis',(1.,0.,0.));
#8554=DIRECTION('center_axis',(0.,-1.,0.));
#8555=DIRECTION('ref_axis',(0.,0.,-1.));
#8556=DIRECTION('center_axis',(0.,1.,0.));
#8557=DIRECTION('ref_axis',(1.,0.,0.));
#8558=DIRECTION('center_axis',(0.,-1.,0.));
#8559=DIRECTION('ref_axis',(1.,0.,0.));
#8560=DIRECTION('center_axis',(0.,-1.,0.));
#8561=DIRECTION('ref_axis',(0.,0.,-1.));
#8562=DIRECTION('center_axis',(6.12323399573676E-17,0.,1.));
#8563=DIRECTION('ref_axis',(1.,0.,0.));
#8564=DIRECTION('center_axis',(0.,-1.,0.));
#8565=DIRECTION('ref_axis',(0.,0.,-1.));
#8566=DIRECTION('center_axis',(0.,1.,0.));
#8567=DIRECTION('ref_axis',(1.,0.,0.));
#8568=DIRECTION('center_axis',(0.,-1.,0.));
#8569=DIRECTION('ref_axis',(1.,0.,0.));
#8570=DIRECTION('center_axis',(0.,-1.,0.));
#8571=DIRECTION('ref_axis',(0.,0.,-1.));
#8572=DIRECTION('center_axis',(0.,0.,1.));
#8573=DIRECTION('ref_axis',(1.,0.,0.));
#8574=DIRECTION('center_axis',(0.,-1.,0.));
#8575=DIRECTION('ref_axis',(0.,0.,-1.));
#8576=DIRECTION('center_axis',(0.,1.,0.));
#8577=DIRECTION('ref_axis',(1.,0.,0.));
#8578=DIRECTION('center_axis',(0.,1.,0.));
#8579=DIRECTION('ref_axis',(1.,0.,0.));
#8580=DIRECTION('',(0.,1.,0.));
#8581=DIRECTION('center_axis',(0.,-1.,0.));
#8582=DIRECTION('ref_axis',(1.,0.,0.));
#8583=DIRECTION('center_axis',(0.,-1.,0.));
#8584=DIRECTION('ref_axis',(1.,0.,0.));
#8585=DIRECTION('center_axis',(0.,1.,0.));
#8586=DIRECTION('ref_axis',(1.,0.,0.));
#8587=DIRECTION('center_axis',(0.,-1.,0.));
#8588=DIRECTION('ref_axis',(0.,0.,-1.));
#8589=DIRECTION('center_axis',(0.,0.,1.));
#8590=DIRECTION('ref_axis',(1.,0.,0.));
#8591=DIRECTION('center_axis',(0.,-1.,0.));
#8592=DIRECTION('ref_axis',(0.,0.,-1.));
#8593=DIRECTION('center_axis',(0.,-1.,0.));
#8594=DIRECTION('ref_axis',(-1.,0.,0.));
#8595=DIRECTION('center_axis',(0.,1.,0.));
#8596=DIRECTION('ref_axis',(1.,0.,0.));
#11188=CARTESIAN_POINT('',(0.,0.,0.));
#11189=CARTESIAN_POINT('Origin',(0.707106781186547,0.,0.707106781186548));
#11190=CARTESIAN_POINT('',(0.504455939115715,-0.04763,0.841298510752802));
#11191=CARTESIAN_POINT('',(0.841298510752802,-0.04763,0.504455939115715));
#11192=CARTESIAN_POINT('Ctrl Pts',(0.504455939115715,-0.04763,0.841298510752802));
#11193=CARTESIAN_POINT('Ctrl Pts',(0.508899795931835,-0.0740444353928835,
0.838633903678357));
#11194=CARTESIAN_POINT('Ctrl Pts',(0.517157748491652,-0.0999305678883309,
0.833661031856294));
#11195=CARTESIAN_POINT('Ctrl Pts',(0.537715343527944,-0.142345102874864,
0.820511285096538));
#11196=CARTESIAN_POINT('Ctrl Pts',(0.548874290046456,-0.159766064500479,
0.813159949759));
#11197=CARTESIAN_POINT('Ctrl Pts',(0.573915184558107,-0.190326085855194,
0.795684265985089));
#11198=CARTESIAN_POINT('Ctrl Pts',(0.587792702767295,-0.203463743702801,
0.78555112003688));
#11199=CARTESIAN_POINT('Ctrl Pts',(0.615966552324775,-0.224161999508995,
0.763642258217233));
#11200=CARTESIAN_POINT('Ctrl Pts',(0.631684198665438,-0.232861760990032,
0.750785745543687));
#11201=CARTESIAN_POINT('Ctrl Pts',(0.663382628119203,-0.244251601209411,
0.722929908501543));
#11202=CARTESIAN_POINT('Ctrl Pts',(0.679352081686668,-0.246942143572133,
0.707917883896095));
#11203=CARTESIAN_POINT('Ctrl Pts',(0.707917883896095,-0.246942143572133,
0.679352081686668));
#11204=CARTESIAN_POINT('Ctrl Pts',(0.722929908501543,-0.244251601209411,
0.663382628119203));
#11205=CARTESIAN_POINT('Ctrl Pts',(0.750785745543687,-0.232861760990032,
0.631684198665439));
#11206=CARTESIAN_POINT('Ctrl Pts',(0.763642258217232,-0.224161999508995,
0.615966552324775));
#11207=CARTESIAN_POINT('Ctrl Pts',(0.78555112003688,-0.203463743702801,
0.587792702767295));
#11208=CARTESIAN_POINT('Ctrl Pts',(0.795684265985088,-0.190326085855194,
0.573915184558108));
#11209=CARTESIAN_POINT('Ctrl Pts',(0.813159949759,-0.15976606450048,0.548874290046456));
#11210=CARTESIAN_POINT('Ctrl Pts',(0.820511285096538,-0.142345102874864,
0.537715343527944));
#11211=CARTESIAN_POINT('Ctrl Pts',(0.833661031856294,-0.099930567888331,
0.517157748491653));
#11212=CARTESIAN_POINT('Ctrl Pts',(0.838633903678357,-0.0740444353928835,
0.508899795931835));
#11213=CARTESIAN_POINT('Ctrl Pts',(0.841298510752801,-0.0476299999999999,
0.504455939115715));
#11214=CARTESIAN_POINT('',(0.528110872004958,-0.04763,0.871530771444223));
#11215=CARTESIAN_POINT('Origin',(0.707106781186547,-0.04763,0.707106781186548));
#11216=CARTESIAN_POINT('',(0.871530771444223,-0.04763,0.528110872004959));
#11217=CARTESIAN_POINT('Ctrl Pts',(0.871530771444223,-0.0476300000000001,
0.528110872004958));
#11218=CARTESIAN_POINT('Ctrl Pts',(0.87014664509073,-0.0609922781173483,
0.530395067942936));
#11219=CARTESIAN_POINT('Ctrl Pts',(0.868149331745851,-0.0742967091364493,
0.533674141594226));
#11220=CARTESIAN_POINT('Ctrl Pts',(0.85981294420286,-0.115492077056649,
0.54708917182331));
#11221=CARTESIAN_POINT('Ctrl Pts',(0.850993704737257,-0.141695629206859,
0.560922177770136));
#11222=CARTESIAN_POINT('Ctrl Pts',(0.830754510485543,-0.181890537957859,
0.590422647829571));
#11223=CARTESIAN_POINT('Ctrl Pts',(0.816896541396381,-0.201072148666545,
0.609616703125488));
#11224=CARTESIAN_POINT('Ctrl Pts',(0.792310597819928,-0.223955109275652,
0.641117951819998));
#11225=CARTESIAN_POINT('Ctrl Pts',(0.779109323683612,-0.232742381310829,
0.657208095763053));
#11226=CARTESIAN_POINT('Ctrl Pts',(0.750552691816206,-0.244234834628584,
0.68964083160521));
#11227=CARTESIAN_POINT('Ctrl Pts',(0.735185187071673,-0.246942143572133,
0.705971972091755));
#11228=CARTESIAN_POINT('Ctrl Pts',(0.705971972091754,-0.246942143572133,
0.735185187071673));
#11229=CARTESIAN_POINT('Ctrl Pts',(0.689640831605209,-0.244234834628584,
0.750552691816206));
#11230=CARTESIAN_POINT('Ctrl Pts',(0.657208095763052,-0.232742381310829,
0.779109323683612));
#11231=CARTESIAN_POINT('Ctrl Pts',(0.641117951819998,-0.223955109275652,
0.792310597819928));
#11232=CARTESIAN_POINT('Ctrl Pts',(0.609616703125487,-0.201072148666545,
0.816896541396382));
#11233=CARTESIAN_POINT('Ctrl Pts',(0.590422647829571,-0.181890537957858,
0.830754510485544));
#11234=CARTESIAN_POINT('Ctrl Pts',(0.560922177770135,-0.141695629206858,
0.850993704737257));
#11235=CARTESIAN_POINT('Ctrl Pts',(0.547089171823309,-0.115492077056649,
0.859812944202861));
#11236=CARTESIAN_POINT('Ctrl Pts',(0.533674141594226,-0.0742967091364491,
0.868149331745852));
#11237=CARTESIAN_POINT('Ctrl Pts',(0.530395067942936,-0.0609922781173483,
0.870146645090731));
#11238=CARTESIAN_POINT('Ctrl Pts',(0.528110872004958,-0.0476300000000001,
0.871530771444223));
#11239=CARTESIAN_POINT('Origin',(0.707106781186547,-0.04763,0.707106781186548));
#11240=CARTESIAN_POINT('Origin',(0.,-0.166705,0.));
#11241=CARTESIAN_POINT('',(0.242834539687906,-0.04763,0.989696097314));
#11242=CARTESIAN_POINT('Origin',(0.,-0.04763,0.));
#11243=CARTESIAN_POINT('',(-0.242834539687907,-0.04763,0.989696097314));
#11244=CARTESIAN_POINT('Ctrl Pts',(0.242834539687906,-0.04763,0.989696097314));
#11245=CARTESIAN_POINT('Ctrl Pts',(0.24024064412003,-0.0609922781173483,
0.990332542620729));
#11246=CARTESIAN_POINT('Ctrl Pts',(0.236509675094874,-0.0742967091364492,
0.991238884025248));
#11247=CARTESIAN_POINT('Ctrl Pts',(0.221129100087819,-0.115492077056649,
0.994830026707808));
#11248=CARTESIAN_POINT('Ctrl Pts',(0.205111543747588,-0.141695629206859,
0.998375294985966));
#11249=CARTESIAN_POINT('Ctrl Pts',(0.169940289819232,-0.181890537957859,
1.00492400591205));
#11250=CARTESIAN_POINT('Ctrl Pts',(0.1465689792446,-0.201072148666545,1.00869718865384));
#11251=CARTESIAN_POINT('Ctrl Pts',(0.106909345252087,-0.223955109275652,
1.01358704779679));
#11252=CARTESIAN_POINT('Ctrl Pts',(0.0861971848975941,-0.232742381310829,
1.0156297872271));
#11253=CARTESIAN_POINT('Ctrl Pts',(0.0430711894098822,-0.244234834628584,
1.01837060663223));
#11254=CARTESIAN_POINT('Ctrl Pts',(0.0206568624125605,-0.246942143572133,
1.019052));
#11255=CARTESIAN_POINT('Ctrl Pts',(-0.0206568624125608,-0.246942143572133,
1.019052));
#11256=CARTESIAN_POINT('Ctrl Pts',(-0.0430711894098825,-0.244234834628584,
1.01837060663223));
#11257=CARTESIAN_POINT('Ctrl Pts',(-0.0861971848975943,-0.232742381310829,
1.0156297872271));
#11258=CARTESIAN_POINT('Ctrl Pts',(-0.106909345252088,-0.223955109275652,
1.01358704779679));
#11259=CARTESIAN_POINT('Ctrl Pts',(-0.1465689792446,-0.201072148666545,
1.00869718865384));
#11260=CARTESIAN_POINT('Ctrl Pts',(-0.169940289819232,-0.181890537957859,
1.00492400591205));
#11261=CARTESIAN_POINT('Ctrl Pts',(-0.205111543747588,-0.141695629206859,
0.998375294985966));
#11262=CARTESIAN_POINT('Ctrl Pts',(-0.221129100087819,-0.115492077056649,
0.994830026707808));
#11263=CARTESIAN_POINT('Ctrl Pts',(-0.236509675094875,-0.0742967091364493,
0.991238884025248));
#11264=CARTESIAN_POINT('Ctrl Pts',(-0.24024064412003,-0.0609922781173483,
0.990332542620729));
#11265=CARTESIAN_POINT('Ctrl Pts',(-0.242834539687907,-0.04763,0.989696097314));
#11266=CARTESIAN_POINT('',(-0.528110872004959,-0.04763,0.871530771444223));
#11267=CARTESIAN_POINT('Origin',(0.,-0.04763,0.));
#11268=CARTESIAN_POINT('',(-0.871530771444223,-0.04763,0.528110872004958));
#11269=CARTESIAN_POINT('Ctrl Pts',(-0.528110872004958,-0.0476300000000001,
0.871530771444223));
#11270=CARTESIAN_POINT('Ctrl Pts',(-0.530395067942936,-0.0609922781173484,
0.87014664509073));
#11271=CARTESIAN_POINT('Ctrl Pts',(-0.533674141594226,-0.0742967091364493,
0.868149331745851));
#11272=CARTESIAN_POINT('Ctrl Pts',(-0.54708917182331,-0.115492077056649,
0.85981294420286));
#11273=CARTESIAN_POINT('Ctrl Pts',(-0.560922177770136,-0.141695629206859,
0.850993704737257));
#11274=CARTESIAN_POINT('Ctrl Pts',(-0.590422647829571,-0.181890537957859,
0.830754510485543));
#11275=CARTESIAN_POINT('Ctrl Pts',(-0.609616703125488,-0.201072148666545,
0.816896541396381));
#11276=CARTESIAN_POINT('Ctrl Pts',(-0.641117951819998,-0.223955109275652,
0.792310597819928));
#11277=CARTESIAN_POINT('Ctrl Pts',(-0.657208095763053,-0.232742381310829,
0.779109323683611));
#11278=CARTESIAN_POINT('Ctrl Pts',(-0.68964083160521,-0.244234834628584,
0.750552691816205));
#11279=CARTESIAN_POINT('Ctrl Pts',(-0.705971972091755,-0.246942143572133,
0.735185187071673));
#11280=CARTESIAN_POINT('Ctrl Pts',(-0.735185187071673,-0.246942143572133,
0.705971972091754));
#11281=CARTESIAN_POINT('Ctrl Pts',(-0.750552691816206,-0.244234834628584,
0.689640831605209));
#11282=CARTESIAN_POINT('Ctrl Pts',(-0.779109323683612,-0.232742381310829,
0.657208095763052));
#11283=CARTESIAN_POINT('Ctrl Pts',(-0.792310597819928,-0.223955109275652,
0.641117951819998));
#11284=CARTESIAN_POINT('Ctrl Pts',(-0.816896541396382,-0.201072148666545,
0.609616703125487));
#11285=CARTESIAN_POINT('Ctrl Pts',(-0.830754510485544,-0.181890537957858,
0.590422647829571));
#11286=CARTESIAN_POINT('Ctrl Pts',(-0.850993704737257,-0.141695629206858,
0.560922177770135));
#11287=CARTESIAN_POINT('Ctrl Pts',(-0.859812944202861,-0.115492077056649,
0.547089171823309));
#11288=CARTESIAN_POINT('Ctrl Pts',(-0.868149331745852,-0.0742967091364491,
0.533674141594226));
#11289=CARTESIAN_POINT('Ctrl Pts',(-0.870146645090731,-0.0609922781173483,
0.530395067942936));
#11290=CARTESIAN_POINT('Ctrl Pts',(-0.871530771444223,-0.04763,0.528110872004958));
#11291=CARTESIAN_POINT('',(-0.989696097314,-0.04763,0.242834539687906));
#11292=CARTESIAN_POINT('Origin',(0.,-0.04763,0.));
#11293=CARTESIAN_POINT('',(-1.019052,-0.246942143572133,1.248489836334E-16));
#11294=CARTESIAN_POINT('Ctrl Pts',(-0.989696097314,-0.04763,0.242834539687906));
#11295=CARTESIAN_POINT('Ctrl Pts',(-0.990332542620729,-0.0609922781173483,
0.24024064412003));
#11296=CARTESIAN_POINT('Ctrl Pts',(-0.991238884025248,-0.0742967091364492,
0.236509675094874));
#11297=CARTESIAN_POINT('Ctrl Pts',(-0.994830026707808,-0.115492077056649,
0.221129100087819));
#11298=CARTESIAN_POINT('Ctrl Pts',(-0.998375294985966,-0.141695629206859,
0.205111543747588));
#11299=CARTESIAN_POINT('Ctrl Pts',(-1.00492400591205,-0.181890537957859,
0.169940289819232));
#11300=CARTESIAN_POINT('Ctrl Pts',(-1.00869718865384,-0.201072148666545,
0.1465689792446));
#11301=CARTESIAN_POINT('Ctrl Pts',(-1.01358704779679,-0.223955109275652,
0.106909345252088));
#11302=CARTESIAN_POINT('Ctrl Pts',(-1.0156297872271,-0.232742381310829,
0.0861971848975944));
#11303=CARTESIAN_POINT('Ctrl Pts',(-1.01837060663223,-0.244234834628584,
0.0430711894098825));
#11304=CARTESIAN_POINT('Ctrl Pts',(-1.019052,-0.246942143572133,0.0206568624125608));
#11305=CARTESIAN_POINT('Ctrl Pts',(-1.019052,-0.246942143572133,1.2490009027033E-16));
#11306=CARTESIAN_POINT('',(-1.019052,-0.28578,1.24797876996471E-16));
#11307=CARTESIAN_POINT('',(-1.019052,-0.166705,1.24797876996471E-16));
#11308=CARTESIAN_POINT('Origin',(0.,-0.28578,0.));
#11309=CARTESIAN_POINT('',(-0.989696097314,-0.04763,-0.242834539687906));
#11310=CARTESIAN_POINT('Ctrl Pts',(-1.019052,-0.246942143572133,1.2490009027033E-16));
#11311=CARTESIAN_POINT('Ctrl Pts',(-1.019052,-0.246942143572133,-0.0206568624125605));
#11312=CARTESIAN_POINT('Ctrl Pts',(-1.01837060663223,-0.244234834628584,
-0.0430711894098822));
#11313=CARTESIAN_POINT('Ctrl Pts',(-1.0156297872271,-0.232742381310829,
-0.0861971848975941));
#11314=CARTESIAN_POINT('Ctrl Pts',(-1.01358704779679,-0.223955109275652,
-0.106909345252087));
#11315=CARTESIAN_POINT('Ctrl Pts',(-1.00869718865384,-0.201072148666546,
-0.1465689792446));
#11316=CARTESIAN_POINT('Ctrl Pts',(-1.00492400591205,-0.181890537957859,
-0.169940289819232));
#11317=CARTESIAN_POINT('Ctrl Pts',(-0.998375294985966,-0.141695629206859,
-0.205111543747588));
#11318=CARTESIAN_POINT('Ctrl Pts',(-0.994830026707808,-0.11549207705665,
-0.221129100087819));
#11319=CARTESIAN_POINT('Ctrl Pts',(-0.991238884025248,-0.0742967091364495,
-0.236509675094874));
#11320=CARTESIAN_POINT('Ctrl Pts',(-0.990332542620729,-0.0609922781173484,
-0.24024064412003));
#11321=CARTESIAN_POINT('Ctrl Pts',(-0.989696097314,-0.0476300000000001,
-0.242834539687907));
#11322=CARTESIAN_POINT('',(-0.871530771444223,-0.04763,-0.528110872004958));
#11323=CARTESIAN_POINT('Origin',(0.,-0.04763,0.));
#11324=CARTESIAN_POINT('',(-0.528110872004958,-0.04763,-0.871530771444223));
#11325=CARTESIAN_POINT('Ctrl Pts',(-0.871530771444223,-0.0476300000000001,
-0.528110872004958));
#11326=CARTESIAN_POINT('Ctrl Pts',(-0.87014664509073,-0.0609922781173484,
-0.530395067942936));
#11327=CARTESIAN_POINT('Ctrl Pts',(-0.868149331745851,-0.0742967091364494,
-0.533674141594226));
#11328=CARTESIAN_POINT('Ctrl Pts',(-0.85981294420286,-0.115492077056649,
-0.54708917182331));
#11329=CARTESIAN_POINT('Ctrl Pts',(-0.850993704737257,-0.141695629206859,
-0.560922177770136));
#11330=CARTESIAN_POINT('Ctrl Pts',(-0.830754510485543,-0.181890537957859,
-0.590422647829571));
#11331=CARTESIAN_POINT('Ctrl Pts',(-0.816896541396381,-0.201072148666546,
-0.609616703125488));
#11332=CARTESIAN_POINT('Ctrl Pts',(-0.792310597819928,-0.223955109275652,
-0.641117951819999));
#11333=CARTESIAN_POINT('Ctrl Pts',(-0.779109323683611,-0.232742381310829,
-0.657208095763053));
#11334=CARTESIAN_POINT('Ctrl Pts',(-0.750552691816205,-0.244234834628584,
-0.68964083160521));
#11335=CARTESIAN_POINT('Ctrl Pts',(-0.735185187071673,-0.246942143572133,
-0.705971972091755));
#11336=CARTESIAN_POINT('Ctrl Pts',(-0.705971972091754,-0.246942143572133,
-0.735185187071673));
#11337=CARTESIAN_POINT('Ctrl Pts',(-0.68964083160521,-0.244234834628584,
-0.750552691816206));
#11338=CARTESIAN_POINT('Ctrl Pts',(-0.657208095763052,-0.232742381310829,
-0.779109323683612));
#11339=CARTESIAN_POINT('Ctrl Pts',(-0.641117951819998,-0.223955109275652,
-0.792310597819928));
#11340=CARTESIAN_POINT('Ctrl Pts',(-0.609616703125488,-0.201072148666545,
-0.816896541396381));
#11341=CARTESIAN_POINT('Ctrl Pts',(-0.590422647829571,-0.181890537957859,
-0.830754510485543));
#11342=CARTESIAN_POINT('Ctrl Pts',(-0.560922177770136,-0.141695629206859,
-0.850993704737257));
#11343=CARTESIAN_POINT('Ctrl Pts',(-0.54708917182331,-0.115492077056649,
-0.85981294420286));
#11344=CARTESIAN_POINT('Ctrl Pts',(-0.533674141594226,-0.0742967091364494,
-0.868149331745852));
#11345=CARTESIAN_POINT('Ctrl Pts',(-0.530395067942936,-0.0609922781173484,
-0.870146645090731));
#11346=CARTESIAN_POINT('Ctrl Pts',(-0.528110872004958,-0.0476300000000001,
-0.871530771444223));
#11347=CARTESIAN_POINT('',(-0.242834539687906,-0.04763,-0.989696097314));
#11348=CARTESIAN_POINT('Origin',(0.,-0.04763,0.));
#11349=CARTESIAN_POINT('',(0.242834539687906,-0.04763,-0.989696097314));
#11350=CARTESIAN_POINT('Ctrl Pts',(-0.242834539687907,-0.04763,-0.989696097314));
#11351=CARTESIAN_POINT('Ctrl Pts',(-0.24024064412003,-0.0609922781173483,
-0.990332542620729));
#11352=CARTESIAN_POINT('Ctrl Pts',(-0.236509675094874,-0.0742967091364493,
-0.991238884025248));
#11353=CARTESIAN_POINT('Ctrl Pts',(-0.221129100087819,-0.115492077056649,
-0.994830026707808));
#11354=CARTESIAN_POINT('Ctrl Pts',(-0.205111543747588,-0.141695629206859,
-0.998375294985966));
#11355=CARTESIAN_POINT('Ctrl Pts',(-0.169940289819232,-0.181890537957859,
-1.00492400591205));
#11356=CARTESIAN_POINT('Ctrl Pts',(-0.1465689792446,-0.201072148666545,
-1.00869718865384));
#11357=CARTESIAN_POINT('Ctrl Pts',(-0.106909345252087,-0.223955109275652,
-1.01358704779679));
#11358=CARTESIAN_POINT('Ctrl Pts',(-0.0861971848975942,-0.232742381310829,
-1.0156297872271));
#11359=CARTESIAN_POINT('Ctrl Pts',(-0.0430711894098823,-0.244234834628584,
-1.01837060663223));
#11360=CARTESIAN_POINT('Ctrl Pts',(-0.0206568624125606,-0.246942143572133,
-1.019052));
#11361=CARTESIAN_POINT('Ctrl Pts',(0.0206568624125607,-0.246942143572133,
-1.019052));
#11362=CARTESIAN_POINT('Ctrl Pts',(0.0430711894098824,-0.244234834628584,
-1.01837060663223));
#11363=CARTESIAN_POINT('Ctrl Pts',(0.0861971848975943,-0.232742381310829,
-1.0156297872271));
#11364=CARTESIAN_POINT('Ctrl Pts',(0.106909345252088,-0.223955109275652,
-1.01358704779679));
#11365=CARTESIAN_POINT('Ctrl Pts',(0.1465689792446,-0.201072148666545,-1.00869718865384));
#11366=CARTESIAN_POINT('Ctrl Pts',(0.169940289819232,-0.181890537957859,
-1.00492400591205));
#11367=CARTESIAN_POINT('Ctrl Pts',(0.205111543747588,-0.141695629206859,
-0.998375294985966));
#11368=CARTESIAN_POINT('Ctrl Pts',(0.221129100087819,-0.115492077056649,
-0.994830026707808));
#11369=CARTESIAN_POINT('Ctrl Pts',(0.236509675094874,-0.0742967091364493,
-0.991238884025248));
#11370=CARTESIAN_POINT('Ctrl Pts',(0.24024064412003,-0.0609922781173484,
-0.990332542620729));
#11371=CARTESIAN_POINT('Ctrl Pts',(0.242834539687907,-0.04763,-0.989696097314));
#11372=CARTESIAN_POINT('',(0.528110872004958,-0.04763,-0.871530771444223));
#11373=CARTESIAN_POINT('Origin',(0.,-0.04763,0.));
#11374=CARTESIAN_POINT('',(0.871530771444223,-0.04763,-0.528110872004958));
#11375=CARTESIAN_POINT('Ctrl Pts',(0.528110872004958,-0.0476300000000001,
-0.871530771444223));
#11376=CARTESIAN_POINT('Ctrl Pts',(0.530395067942936,-0.0609922781173484,
-0.870146645090731));
#11377=CARTESIAN_POINT('Ctrl Pts',(0.533674141594226,-0.0742967091364493,
-0.868149331745851));
#11378=CARTESIAN_POINT('Ctrl Pts',(0.54708917182331,-0.115492077056649,
-0.85981294420286));
#11379=CARTESIAN_POINT('Ctrl Pts',(0.560922177770136,-0.141695629206859,
-0.850993704737257));
#11380=CARTESIAN_POINT('Ctrl Pts',(0.590422647829571,-0.181890537957859,
-0.830754510485543));
#11381=CARTESIAN_POINT('Ctrl Pts',(0.609616703125488,-0.201072148666545,
-0.816896541396381));
#11382=CARTESIAN_POINT('Ctrl Pts',(0.641117951819998,-0.223955109275652,
-0.792310597819928));
#11383=CARTESIAN_POINT('Ctrl Pts',(0.657208095763053,-0.232742381310829,
-0.779109323683612));
#11384=CARTESIAN_POINT('Ctrl Pts',(0.68964083160521,-0.244234834628584,
-0.750552691816206));
#11385=CARTESIAN_POINT('Ctrl Pts',(0.705971972091755,-0.246942143572133,
-0.735185187071673));
#11386=CARTESIAN_POINT('Ctrl Pts',(0.735185187071673,-0.246942143572133,
-0.705971972091754));
#11387=CARTESIAN_POINT('Ctrl Pts',(0.750552691816206,-0.244234834628584,
-0.68964083160521));
#11388=CARTESIAN_POINT('Ctrl Pts',(0.779109323683612,-0.232742381310829,
-0.657208095763053));
#11389=CARTESIAN_POINT('Ctrl Pts',(0.792310597819928,-0.223955109275652,
-0.641117951819998));
#11390=CARTESIAN_POINT('Ctrl Pts',(0.816896541396381,-0.201072148666545,
-0.609616703125488));
#11391=CARTESIAN_POINT('Ctrl Pts',(0.830754510485543,-0.181890537957859,
-0.590422647829571));
#11392=CARTESIAN_POINT('Ctrl Pts',(0.850993704737257,-0.141695629206859,
-0.560922177770136));
#11393=CARTESIAN_POINT('Ctrl Pts',(0.85981294420286,-0.115492077056649,
-0.54708917182331));
#11394=CARTESIAN_POINT('Ctrl Pts',(0.868149331745851,-0.0742967091364493,
-0.533674141594226));
#11395=CARTESIAN_POINT('Ctrl Pts',(0.870146645090731,-0.0609922781173484,
-0.530395067942936));
#11396=CARTESIAN_POINT('Ctrl Pts',(0.871530771444223,-0.0476300000000001,
-0.528110872004958));
#11397=CARTESIAN_POINT('',(0.989696097314,-0.04763,-0.242834539687906));
#11398=CARTESIAN_POINT('Origin',(0.,-0.04763,0.));
#11399=CARTESIAN_POINT('',(0.989696097314,-0.04763,0.242834539687906));
#11400=CARTESIAN_POINT('Ctrl Pts',(0.989696097314,-0.04763,-0.242834539687907));
#11401=CARTESIAN_POINT('Ctrl Pts',(0.990332542620729,-0.0609922781173483,
-0.24024064412003));
#11402=CARTESIAN_POINT('Ctrl Pts',(0.991238884025248,-0.0742967091364493,
-0.236509675094874));
#11403=CARTESIAN_POINT('Ctrl Pts',(0.994830026707808,-0.115492077056649,
-0.221129100087819));
#11404=CARTESIAN_POINT('Ctrl Pts',(0.998375294985966,-0.141695629206859,
-0.205111543747588));
#11405=CARTESIAN_POINT('Ctrl Pts',(1.00492400591205,-0.181890537957859,
-0.169940289819232));
#11406=CARTESIAN_POINT('Ctrl Pts',(1.00869718865384,-0.201072148666545,
-0.1465689792446));
#11407=CARTESIAN_POINT('Ctrl Pts',(1.01358704779679,-0.223955109275652,
-0.106909345252087));
#11408=CARTESIAN_POINT('Ctrl Pts',(1.0156297872271,-0.232742381310829,-0.0861971848975942));
#11409=CARTESIAN_POINT('Ctrl Pts',(1.01837060663223,-0.244234834628584,
-0.0430711894098823));
#11410=CARTESIAN_POINT('Ctrl Pts',(1.019052,-0.246942143572133,-0.0206568624125607));
#11411=CARTESIAN_POINT('Ctrl Pts',(1.019052,-0.246942143572133,0.0206568624125607));
#11412=CARTESIAN_POINT('Ctrl Pts',(1.01837060663223,-0.244234834628584,
0.0430711894098823));
#11413=CARTESIAN_POINT('Ctrl Pts',(1.0156297872271,-0.232742381310829,0.0861971848975942));
#11414=CARTESIAN_POINT('Ctrl Pts',(1.01358704779679,-0.223955109275652,
0.106909345252087));
#11415=CARTESIAN_POINT('Ctrl Pts',(1.00869718865384,-0.201072148666545,
0.1465689792446));
#11416=CARTESIAN_POINT('Ctrl Pts',(1.00492400591205,-0.181890537957859,
0.169940289819232));
#11417=CARTESIAN_POINT('Ctrl Pts',(0.998375294985966,-0.141695629206859,
0.205111543747588));
#11418=CARTESIAN_POINT('Ctrl Pts',(0.994830026707808,-0.115492077056649,
0.221129100087819));
#11419=CARTESIAN_POINT('Ctrl Pts',(0.991238884025248,-0.0742967091364492,
0.236509675094874));
#11420=CARTESIAN_POINT('Ctrl Pts',(0.990332542620729,-0.0609922781173483,
0.24024064412003));
#11421=CARTESIAN_POINT('Ctrl Pts',(0.989696097314,-0.04763,0.242834539687907));
#11422=CARTESIAN_POINT('Origin',(0.,-0.04763,0.));
#11423=CARTESIAN_POINT('Origin',(0.,-0.04763,0.));
#11424=CARTESIAN_POINT('',(0.238183666596899,-0.04763,0.951592097314));
#11425=CARTESIAN_POINT('Origin',(0.,-0.04763,0.));
#11426=CARTESIAN_POINT('Origin',(-1.94289029309402E-16,-0.04763,1.));
#11427=CARTESIAN_POINT('Origin',(-1.94289029309402E-16,0.,1.));
#11428=CARTESIAN_POINT('',(-0.2381836665969,-0.04763,0.951592097314));
#11429=CARTESIAN_POINT('Ctrl Pts',(-0.238183666596899,-0.0476299999999999,
0.951592097314));
#11430=CARTESIAN_POINT('Ctrl Pts',(-0.233157223576062,-0.0740444353928835,
0.952850216871763));
#11431=CARTESIAN_POINT('Ctrl Pts',(-0.223801617934946,-0.0999305678883309,
0.955173119738174));
#11432=CARTESIAN_POINT('Ctrl Pts',(-0.199966927975188,-0.142345102874864,
0.960411259488514));
#11433=CARTESIAN_POINT('Ctrl Pts',(-0.1868781821531,-0.159766064500479,
0.963103647174702));
#11434=CARTESIAN_POINT('Ctrl Pts',(-0.15681442133453,-0.190326085855194,
0.968453058988463));
#11435=CARTESIAN_POINT('Ctrl Pts',(-0.139836317888043,-0.203463743702801,
0.971100730005489));
#11436=CARTESIAN_POINT('Ctrl Pts',(-0.104422493053067,-0.224161999508995,
0.975530745318961));
#11437=CARTESIAN_POINT('Ctrl Pts',(-0.0842175114474176,-0.232861760990032,
0.977553872336861));
#11438=CARTESIAN_POINT('Ctrl Pts',(-0.0421062857595701,-0.244251601209411,
0.980270995488453));
#11439=CARTESIAN_POINT('Ctrl Pts',(-0.0201990724523197,-0.246942143572133,
0.980948));
#11440=CARTESIAN_POINT('Ctrl Pts',(0.020199072452319,-0.246942143572133,
0.980948));
#11441=CARTESIAN_POINT('Ctrl Pts',(0.0421062857595694,-0.244251601209411,
0.980270995488454));
#11442=CARTESIAN_POINT('Ctrl Pts',(0.0842175114474169,-0.232861760990032,
0.977553872336861));
#11443=CARTESIAN_POINT('Ctrl Pts',(0.104422493053067,-0.224161999508995,
0.975530745318961));
#11444=CARTESIAN_POINT('Ctrl Pts',(0.139836317888042,-0.203463743702801,
0.971100730005489));
#11445=CARTESIAN_POINT('Ctrl Pts',(0.15681442133453,-0.190326085855194,
0.968453058988463));
#11446=CARTESIAN_POINT('Ctrl Pts',(0.1868781821531,-0.15976606450048,0.963103647174702));
#11447=CARTESIAN_POINT('Ctrl Pts',(0.199966927975188,-0.142345102874864,
0.960411259488514));
#11448=CARTESIAN_POINT('Ctrl Pts',(0.223801617934945,-0.0999305678883309,
0.955173119738174));
#11449=CARTESIAN_POINT('Ctrl Pts',(0.233157223576061,-0.0740444353928835,
0.952850216871763));
#11450=CARTESIAN_POINT('Ctrl Pts',(0.238183666596899,-0.0476299999999999,
0.951592097314));
#11451=CARTESIAN_POINT('Origin',(-1.94289029309402E-16,-0.04763,1.));
#11452=CARTESIAN_POINT('Origin',(0.,-0.04763,0.));
#11453=CARTESIAN_POINT('',(-0.504455939115715,-0.04763,0.841298510752802));
#11454=CARTESIAN_POINT('Origin',(0.,-0.04763,0.));
#11455=CARTESIAN_POINT('Origin',(-0.707106781186548,-0.04763,0.707106781186547));
#11456=CARTESIAN_POINT('Origin',(-0.707106781186548,0.,0.707106781186547));
#11457=CARTESIAN_POINT('',(-0.841298510752802,-0.04763,0.504455939115715));
#11458=CARTESIAN_POINT('Ctrl Pts',(-0.841298510752802,-0.04763,0.504455939115715));
#11459=CARTESIAN_POINT('Ctrl Pts',(-0.838633903678357,-0.0740444353928835,
0.508899795931835));
#11460=CARTESIAN_POINT('Ctrl Pts',(-0.833661031856294,-0.0999305678883309,
0.517157748491652));
#11461=CARTESIAN_POINT('Ctrl Pts',(-0.820511285096538,-0.142345102874864,
0.537715343527944));
#11462=CARTESIAN_POINT('Ctrl Pts',(-0.813159949759,-0.159766064500479,0.548874290046456));
#11463=CARTESIAN_POINT('Ctrl Pts',(-0.795684265985089,-0.190326085855194,
0.573915184558107));
#11464=CARTESIAN_POINT('Ctrl Pts',(-0.78555112003688,-0.203463743702801,
0.587792702767295));
#11465=CARTESIAN_POINT('Ctrl Pts',(-0.763642258217233,-0.224161999508995,
0.615966552324775));
#11466=CARTESIAN_POINT('Ctrl Pts',(-0.750785745543687,-0.232861760990032,
0.631684198665438));
#11467=CARTESIAN_POINT('Ctrl Pts',(-0.722929908501543,-0.244251601209411,
0.663382628119203));
#11468=CARTESIAN_POINT('Ctrl Pts',(-0.707917883896095,-0.246942143572133,
0.679352081686668));
#11469=CARTESIAN_POINT('Ctrl Pts',(-0.679352081686668,-0.246942143572133,
0.707917883896095));
#11470=CARTESIAN_POINT('Ctrl Pts',(-0.663382628119203,-0.244251601209411,
0.722929908501544));
#11471=CARTESIAN_POINT('Ctrl Pts',(-0.631684198665438,-0.232861760990031,
0.750785745543687));
#11472=CARTESIAN_POINT('Ctrl Pts',(-0.615966552324775,-0.224161999508995,
0.763642258217233));
#11473=CARTESIAN_POINT('Ctrl Pts',(-0.587792702767295,-0.203463743702801,
0.78555112003688));
#11474=CARTESIAN_POINT('Ctrl Pts',(-0.573915184558107,-0.190326085855194,
0.795684265985088));
#11475=CARTESIAN_POINT('Ctrl Pts',(-0.548874290046456,-0.159766064500479,
0.813159949759));
#11476=CARTESIAN_POINT('Ctrl Pts',(-0.537715343527944,-0.142345102874864,
0.820511285096538));
#11477=CARTESIAN_POINT('Ctrl Pts',(-0.517157748491652,-0.0999305678883309,
0.833661031856294));
#11478=CARTESIAN_POINT('Ctrl Pts',(-0.508899795931835,-0.0740444353928835,
0.838633903678357));
#11479=CARTESIAN_POINT('Ctrl Pts',(-0.504455939115716,-0.04763,0.841298510752801));
#11480=CARTESIAN_POINT('Origin',(-0.707106781186548,-0.04763,0.707106781186547));
#11481=CARTESIAN_POINT('Origin',(0.,-0.04763,0.));
#11482=CARTESIAN_POINT('',(-0.951592097314,-0.04763,0.238183666596899));
#11483=CARTESIAN_POINT('Origin',(0.,-0.04763,0.));
#11484=CARTESIAN_POINT('Origin',(-1.,-0.04763,-1.11022302462516E-16));
#11485=CARTESIAN_POINT('Origin',(-1.,0.,-1.11022302462516E-16));
#11486=CARTESIAN_POINT('',(-0.951592097314,-0.04763,-0.2381836665969));
#11487=CARTESIAN_POINT('',(-0.980948,-0.246942143572133,1.08514323328844E-18));
#11488=CARTESIAN_POINT('Ctrl Pts',(-0.951592097314,-0.04763,-0.238183666596899));
#11489=CARTESIAN_POINT('Ctrl Pts',(-0.952850216871763,-0.0740444353928835,
-0.233157223576062));
#11490=CARTESIAN_POINT('Ctrl Pts',(-0.955173119738174,-0.0999305678883309,
-0.223801617934946));
#11491=CARTESIAN_POINT('Ctrl Pts',(-0.960411259488514,-0.142345102874864,
-0.199966927975188));
#11492=CARTESIAN_POINT('Ctrl Pts',(-0.963103647174702,-0.159766064500479,
-0.1868781821531));
#11493=CARTESIAN_POINT('Ctrl Pts',(-0.968453058988463,-0.190326085855194,
-0.15681442133453));
#11494=CARTESIAN_POINT('Ctrl Pts',(-0.971100730005489,-0.203463743702801,
-0.139836317888043));
#11495=CARTESIAN_POINT('Ctrl Pts',(-0.975530745318961,-0.224161999508995,
-0.104422493053067));
#11496=CARTESIAN_POINT('Ctrl Pts',(-0.977553872336861,-0.232861760990032,
-0.0842175114474175));
#11497=CARTESIAN_POINT('Ctrl Pts',(-0.980270995488453,-0.244251601209411,
-0.0421062857595699));
#11498=CARTESIAN_POINT('Ctrl Pts',(-0.980948,-0.246942143572133,-0.0201990724523195));
#11499=CARTESIAN_POINT('Ctrl Pts',(-0.980948,-0.246942143572133,-1.17961196366423E-16));
#11500=CARTESIAN_POINT('Origin',(-1.,-0.04763,-1.11022302462516E-16));
#11501=CARTESIAN_POINT('Ctrl Pts',(-0.980948,-0.246942143572133,-1.17961196366423E-16));
#11502=CARTESIAN_POINT('Ctrl Pts',(-0.980948,-0.246942143572133,0.0201990724523192));
#11503=CARTESIAN_POINT('Ctrl Pts',(-0.980270995488453,-0.244251601209411,
0.0421062857595695));
#11504=CARTESIAN_POINT('Ctrl Pts',(-0.977553872336861,-0.232861760990032,
0.0842175114474169));
#11505=CARTESIAN_POINT('Ctrl Pts',(-0.975530745318961,-0.224161999508995,
0.104422493053066));
#11506=CARTESIAN_POINT('Ctrl Pts',(-0.971100730005489,-0.203463743702801,
0.139836317888042));
#11507=CARTESIAN_POINT('Ctrl Pts',(-0.968453058988463,-0.190326085855194,
0.15681442133453));
#11508=CARTESIAN_POINT('Ctrl Pts',(-0.963103647174702,-0.15976606450048,
0.1868781821531));
#11509=CARTESIAN_POINT('Ctrl Pts',(-0.960411259488514,-0.142345102874864,
0.199966927975188));
#11510=CARTESIAN_POINT('Ctrl Pts',(-0.955173119738174,-0.099930567888331,
0.223801617934945));
#11511=CARTESIAN_POINT('Ctrl Pts',(-0.952850216871763,-0.0740444353928835,
0.233157223576061));
#11512=CARTESIAN_POINT('Ctrl Pts',(-0.951592097314,-0.04763,0.238183666596899));
#11513=CARTESIAN_POINT('Origin',(0.,-0.04763,0.));
#11514=CARTESIAN_POINT('',(-0.841298510752802,-0.04763,-0.504455939115715));
#11515=CARTESIAN_POINT('Origin',(0.,-0.04763,0.));
#11516=CARTESIAN_POINT('Origin',(-0.707106781186547,-0.04763,-0.707106781186548));
#11517=CARTESIAN_POINT('Origin',(-0.707106781186547,0.,-0.707106781186548));
#11518=CARTESIAN_POINT('',(-0.504455939115715,-0.04763,-0.841298510752802));
#11519=CARTESIAN_POINT('Ctrl Pts',(-0.504455939115715,-0.04763,-0.841298510752802));
#11520=CARTESIAN_POINT('Ctrl Pts',(-0.508899795931835,-0.0740444353928835,
-0.838633903678357));
#11521=CARTESIAN_POINT('Ctrl Pts',(-0.517157748491652,-0.0999305678883309,
-0.833661031856294));
#11522=CARTESIAN_POINT('Ctrl Pts',(-0.537715343527944,-0.142345102874864,
-0.820511285096538));
#11523=CARTESIAN_POINT('Ctrl Pts',(-0.548874290046456,-0.159766064500479,
-0.813159949759));
#11524=CARTESIAN_POINT('Ctrl Pts',(-0.573915184558107,-0.190326085855194,
-0.795684265985089));
#11525=CARTESIAN_POINT('Ctrl Pts',(-0.587792702767295,-0.203463743702801,
-0.78555112003688));
#11526=CARTESIAN_POINT('Ctrl Pts',(-0.615966552324775,-0.224161999508995,
-0.763642258217233));
#11527=CARTESIAN_POINT('Ctrl Pts',(-0.631684198665438,-0.232861760990032,
-0.750785745543687));
#11528=CARTESIAN_POINT('Ctrl Pts',(-0.663382628119203,-0.244251601209411,
-0.722929908501543));
#11529=CARTESIAN_POINT('Ctrl Pts',(-0.679352081686668,-0.246942143572133,
-0.707917883896095));
#11530=CARTESIAN_POINT('Ctrl Pts',(-0.707917883896095,-0.246942143572133,
-0.679352081686668));
#11531=CARTESIAN_POINT('Ctrl Pts',(-0.722929908501543,-0.244251601209411,
-0.663382628119203));
#11532=CARTESIAN_POINT('Ctrl Pts',(-0.750785745543687,-0.232861760990032,
-0.631684198665439));
#11533=CARTESIAN_POINT('Ctrl Pts',(-0.763642258217232,-0.224161999508995,
-0.615966552324775));
#11534=CARTESIAN_POINT('Ctrl Pts',(-0.78555112003688,-0.203463743702801,
-0.587792702767295));
#11535=CARTESIAN_POINT('Ctrl Pts',(-0.795684265985088,-0.190326085855194,
-0.573915184558107));
#11536=CARTESIAN_POINT('Ctrl Pts',(-0.813159949759,-0.15976606450048,-0.548874290046456));
#11537=CARTESIAN_POINT('Ctrl Pts',(-0.820511285096538,-0.142345102874864,
-0.537715343527944));
#11538=CARTESIAN_POINT('Ctrl Pts',(-0.833661031856294,-0.0999305678883311,
-0.517157748491652));
#11539=CARTESIAN_POINT('Ctrl Pts',(-0.838633903678357,-0.0740444353928836,
-0.508899795931835));
#11540=CARTESIAN_POINT('Ctrl Pts',(-0.841298510752801,-0.04763,-0.504455939115715));
#11541=CARTESIAN_POINT('Origin',(-0.707106781186547,-0.04763,-0.707106781186548));
#11542=CARTESIAN_POINT('Origin',(0.,-0.04763,0.));
#11543=CARTESIAN_POINT('',(-0.238183666596899,-0.04763,-0.951592097314));
#11544=CARTESIAN_POINT('Origin',(0.,-0.04763,0.));
#11545=CARTESIAN_POINT('Origin',(5.55111512312578E-17,-0.04763,-1.));
#11546=CARTESIAN_POINT('Origin',(5.55111512312578E-17,0.,-1.));
#11547=CARTESIAN_POINT('',(0.238183666596899,-0.04763,-0.951592097314));
#11548=CARTESIAN_POINT('Ctrl Pts',(0.238183666596899,-0.04763,-0.951592097314));
#11549=CARTESIAN_POINT('Ctrl Pts',(0.233157223576062,-0.0740444353928835,
-0.952850216871763));
#11550=CARTESIAN_POINT('Ctrl Pts',(0.223801617934946,-0.099930567888331,
-0.955173119738174));
#11551=CARTESIAN_POINT('Ctrl Pts',(0.199966927975188,-0.142345102874864,
-0.960411259488514));
#11552=CARTESIAN_POINT('Ctrl Pts',(0.1868781821531,-0.15976606450048,-0.963103647174702));
#11553=CARTESIAN_POINT('Ctrl Pts',(0.15681442133453,-0.190326085855194,
-0.968453058988463));
#11554=CARTESIAN_POINT('Ctrl Pts',(0.139836317888042,-0.203463743702801,
-0.971100730005489));
#11555=CARTESIAN_POINT('Ctrl Pts',(0.104422493053067,-0.224161999508995,
-0.975530745318961));
#11556=CARTESIAN_POINT('Ctrl Pts',(0.0842175114474173,-0.232861760990032,
-0.977553872336861));
#11557=CARTESIAN_POINT('Ctrl Pts',(0.0421062857595698,-0.244251601209411,
-0.980270995488453));
#11558=CARTESIAN_POINT('Ctrl Pts',(0.0201990724523194,-0.246942143572133,
-0.980948));
#11559=CARTESIAN_POINT('Ctrl Pts',(-0.0201990724523193,-0.246942143572133,
-0.980948));
#11560=CARTESIAN_POINT('Ctrl Pts',(-0.0421062857595697,-0.244251601209411,
-0.980270995488453));
#11561=CARTESIAN_POINT('Ctrl Pts',(-0.0842175114474171,-0.232861760990032,
-0.977553872336861));
#11562=CARTESIAN_POINT('Ctrl Pts',(-0.104422493053067,-0.224161999508995,
-0.975530745318961));
#11563=CARTESIAN_POINT('Ctrl Pts',(-0.139836317888042,-0.203463743702801,
-0.971100730005489));
#11564=CARTESIAN_POINT('Ctrl Pts',(-0.15681442133453,-0.190326085855194,
-0.968453058988463));
#11565=CARTESIAN_POINT('Ctrl Pts',(-0.1868781821531,-0.15976606450048,-0.963103647174702));
#11566=CARTESIAN_POINT('Ctrl Pts',(-0.199966927975188,-0.142345102874864,
-0.960411259488514));
#11567=CARTESIAN_POINT('Ctrl Pts',(-0.223801617934945,-0.099930567888331,
-0.955173119738174));
#11568=CARTESIAN_POINT('Ctrl Pts',(-0.233157223576062,-0.0740444353928835,
-0.952850216871763));
#11569=CARTESIAN_POINT('Ctrl Pts',(-0.238183666596899,-0.0476299999999999,
-0.951592097314));
#11570=CARTESIAN_POINT('Origin',(5.55111512312578E-17,-0.04763,-1.));
#11571=CARTESIAN_POINT('Origin',(0.,-0.04763,0.));
#11572=CARTESIAN_POINT('',(0.504455939115715,-0.04763,-0.841298510752802));
#11573=CARTESIAN_POINT('Origin',(0.,-0.04763,0.));
#11574=CARTESIAN_POINT('Origin',(0.707106781186548,-0.04763,-0.707106781186547));
#11575=CARTESIAN_POINT('Origin',(0.707106781186548,0.,-0.707106781186547));
#11576=CARTESIAN_POINT('',(0.841298510752802,-0.04763,-0.504455939115715));
#11577=CARTESIAN_POINT('Ctrl Pts',(0.841298510752802,-0.04763,-0.504455939115715));
#11578=CARTESIAN_POINT('Ctrl Pts',(0.838633903678357,-0.0740444353928835,
-0.508899795931835));
#11579=CARTESIAN_POINT('Ctrl Pts',(0.833661031856294,-0.0999305678883309,
-0.517157748491652));
#11580=CARTESIAN_POINT('Ctrl Pts',(0.820511285096538,-0.142345102874864,
-0.537715343527944));
#11581=CARTESIAN_POINT('Ctrl Pts',(0.813159949759,-0.159766064500479,-0.548874290046456));
#11582=CARTESIAN_POINT('Ctrl Pts',(0.795684265985088,-0.190326085855194,
-0.573915184558107));
#11583=CARTESIAN_POINT('Ctrl Pts',(0.78555112003688,-0.203463743702801,
-0.587792702767295));
#11584=CARTESIAN_POINT('Ctrl Pts',(0.763642258217233,-0.224161999508995,
-0.615966552324775));
#11585=CARTESIAN_POINT('Ctrl Pts',(0.750785745543687,-0.232861760990032,
-0.631684198665438));
#11586=CARTESIAN_POINT('Ctrl Pts',(0.722929908501543,-0.244251601209411,
-0.663382628119203));
#11587=CARTESIAN_POINT('Ctrl Pts',(0.707917883896095,-0.246942143572133,
-0.679352081686668));
#11588=CARTESIAN_POINT('Ctrl Pts',(0.679352081686668,-0.246942143572133,
-0.707917883896095));
#11589=CARTESIAN_POINT('Ctrl Pts',(0.663382628119203,-0.244251601209411,
-0.722929908501543));
#11590=CARTESIAN_POINT('Ctrl Pts',(0.631684198665438,-0.232861760990032,
-0.750785745543687));
#11591=CARTESIAN_POINT('Ctrl Pts',(0.615966552324775,-0.224161999508995,
-0.763642258217232));
#11592=CARTESIAN_POINT('Ctrl Pts',(0.587792702767295,-0.203463743702801,
-0.78555112003688));
#11593=CARTESIAN_POINT('Ctrl Pts',(0.573915184558107,-0.190326085855194,
-0.795684265985088));
#11594=CARTESIAN_POINT('Ctrl Pts',(0.548874290046456,-0.159766064500479,
-0.813159949759));
#11595=CARTESIAN_POINT('Ctrl Pts',(0.537715343527944,-0.142345102874864,
-0.820511285096538));
#11596=CARTESIAN_POINT('Ctrl Pts',(0.517157748491652,-0.099930567888331,
-0.833661031856294));
#11597=CARTESIAN_POINT('Ctrl Pts',(0.508899795931835,-0.0740444353928835,
-0.838633903678357));
#11598=CARTESIAN_POINT('Ctrl Pts',(0.504455939115715,-0.04763,-0.841298510752801));
#11599=CARTESIAN_POINT('Origin',(0.707106781186548,-0.04763,-0.707106781186547));
#11600=CARTESIAN_POINT('Origin',(0.,-0.166705,0.));
#11601=CARTESIAN_POINT('',(-0.980948,-0.28578,1.20131482833E-16));
#11602=CARTESIAN_POINT('Origin',(0.,-0.28578,0.));
#11603=CARTESIAN_POINT('',(-0.980948,-0.166705,1.20131482833E-16));
#11604=CARTESIAN_POINT('',(0.951592097314,-0.04763,0.238183666596899));
#11605=CARTESIAN_POINT('Origin',(0.,-0.04763,0.));
#11606=CARTESIAN_POINT('',(0.951592097314,-0.04763,-0.238183666596899));
#11607=CARTESIAN_POINT('Ctrl Pts',(0.951592097314,-0.04763,0.238183666596899));
#11608=CARTESIAN_POINT('Ctrl Pts',(0.952850216871763,-0.0740444353928835,
0.233157223576062));
#11609=CARTESIAN_POINT('Ctrl Pts',(0.955173119738174,-0.099930567888331,
0.223801617934945));
#11610=CARTESIAN_POINT('Ctrl Pts',(0.960411259488514,-0.142345102874864,
0.199966927975188));
#11611=CARTESIAN_POINT('Ctrl Pts',(0.963103647174702,-0.15976606450048,
0.1868781821531));
#11612=CARTESIAN_POINT('Ctrl Pts',(0.968453058988463,-0.190326085855194,
0.15681442133453));
#11613=CARTESIAN_POINT('Ctrl Pts',(0.971100730005489,-0.203463743702801,
0.139836317888042));
#11614=CARTESIAN_POINT('Ctrl Pts',(0.975530745318961,-0.224161999508995,
0.104422493053067));
#11615=CARTESIAN_POINT('Ctrl Pts',(0.977553872336861,-0.232861760990032,
0.0842175114474172));
#11616=CARTESIAN_POINT('Ctrl Pts',(0.980270995488453,-0.244251601209411,
0.0421062857595697));
#11617=CARTESIAN_POINT('Ctrl Pts',(0.980948,-0.246942143572133,0.0201990724523194));
#11618=CARTESIAN_POINT('Ctrl Pts',(0.980948,-0.246942143572133,-0.0201990724523194));
#11619=CARTESIAN_POINT('Ctrl Pts',(0.980270995488453,-0.244251601209411,
-0.0421062857595697));
#11620=CARTESIAN_POINT('Ctrl Pts',(0.977553872336861,-0.232861760990032,
-0.0842175114474172));
#11621=CARTESIAN_POINT('Ctrl Pts',(0.975530745318961,-0.224161999508995,
-0.104422493053067));
#11622=CARTESIAN_POINT('Ctrl Pts',(0.971100730005489,-0.203463743702801,
-0.139836317888042));
#11623=CARTESIAN_POINT('Ctrl Pts',(0.968453058988463,-0.190326085855194,
-0.15681442133453));
#11624=CARTESIAN_POINT('Ctrl Pts',(0.963103647174702,-0.15976606450048,
-0.1868781821531));
#11625=CARTESIAN_POINT('Ctrl Pts',(0.960411259488514,-0.142345102874864,
-0.199966927975188));
#11626=CARTESIAN_POINT('Ctrl Pts',(0.955173119738174,-0.099930567888331,
-0.223801617934945));
#11627=CARTESIAN_POINT('Ctrl Pts',(0.952850216871763,-0.0740444353928835,
-0.233157223576062));
#11628=CARTESIAN_POINT('Ctrl Pts',(0.951592097314,-0.0476299999999999,-0.238183666596899));
#11629=CARTESIAN_POINT('Origin',(0.,-0.04763,0.));
#11630=CARTESIAN_POINT('Origin',(0.,-0.04763,0.));
#11631=CARTESIAN_POINT('Origin',(1.,-0.04763,0.));
#11632=CARTESIAN_POINT('Origin',(1.,0.,0.));
#11633=CARTESIAN_POINT('Origin',(1.,-0.04763,0.));
#11634=CARTESIAN_POINT('Origin',(0.,-0.28578,0.));
#11635=CARTESIAN_POINT('Origin',(0.,-0.04763,0.));
#12725=UNCERTAINTY_MEASURE_WITH_UNIT(LENGTH_MEASURE(0.001),#12780,
'DISTANCE_ACCURACY_VALUE',
'Maximum model space distance between geometric entities at asserted c
onnectivities');
#12739=UNCERTAINTY_MEASURE_WITH_UNIT(LENGTH_MEASURE(0.001),#12780,
'DISTANCE_ACCURACY_VALUE',
'Maximum model space distance between geometric entities at asserted c
onnectivities');
#12765=(
GEOMETRIC_REPRESENTATION_CONTEXT(3)
GLOBAL_UNCERTAINTY_ASSIGNED_CONTEXT((#12725))
GLOBAL_UNIT_ASSIGNED_CONTEXT((#12780,#12782,#12783))
REPRESENTATION_CONTEXT('','3D')
);
#12779=(
GEOMETRIC_REPRESENTATION_CONTEXT(3)
GLOBAL_UNCERTAINTY_ASSIGNED_CONTEXT((#12739))
GLOBAL_UNIT_ASSIGNED_CONTEXT((#12780,#12782,#12783))
REPRESENTATION_CONTEXT('','3D')
);
#12780=(
LENGTH_UNIT()
NAMED_UNIT(*)
SI_UNIT(.CENTI.,.METRE.)
);
#12782=(
NAMED_UNIT(*)
PLANE_ANGLE_UNIT()
SI_UNIT($,.RADIAN.)
);
#12783=(
NAMED_UNIT(*)
SI_UNIT($,.STERADIAN.)
SOLID_ANGLE_UNIT()
);
#12809=SHAPE_DEFINITION_REPRESENTATION(#12848,#12948);
#12848=PRODUCT_DEFINITION_SHAPE('',$,#12988);
#12948=SHAPE_REPRESENTATION('',(#7024),#12765);
#12962=PRODUCT_DEFINITION_CONTEXT('part definition',#13081,'design');
#12988=PRODUCT_DEFINITION('Cage','Cage',#13027,#12962);
#13027=PRODUCT_DEFINITION_FORMATION('',$,#13108);
#13081=APPLICATION_CONTEXT(
'Core Data for Automotive Mechanical Design Process');
#13082=PRODUCT_CONTEXT('part definition',#13081,'mechanical');
#13108=PRODUCT('Cage','Cage','Cage',(#13082));
#13178=COLOUR_RGB('Grey',0.48,0.52,0.57);
#13179=FILL_AREA_STYLE_COLOUR('',#13178);
#13180=FILL_AREA_STYLE('',(#13179));
#13181=SURFACE_STYLE_FILL_AREA(#13180);
#13182=SURFACE_SIDE_STYLE('',(#13181));
#13183=SURFACE_STYLE_USAGE(.BOTH.,#13182);
#13184=PRESENTATION_STYLE_ASSIGNMENT((#13183));
ENDSEC;
END-ISO-10303-21;
